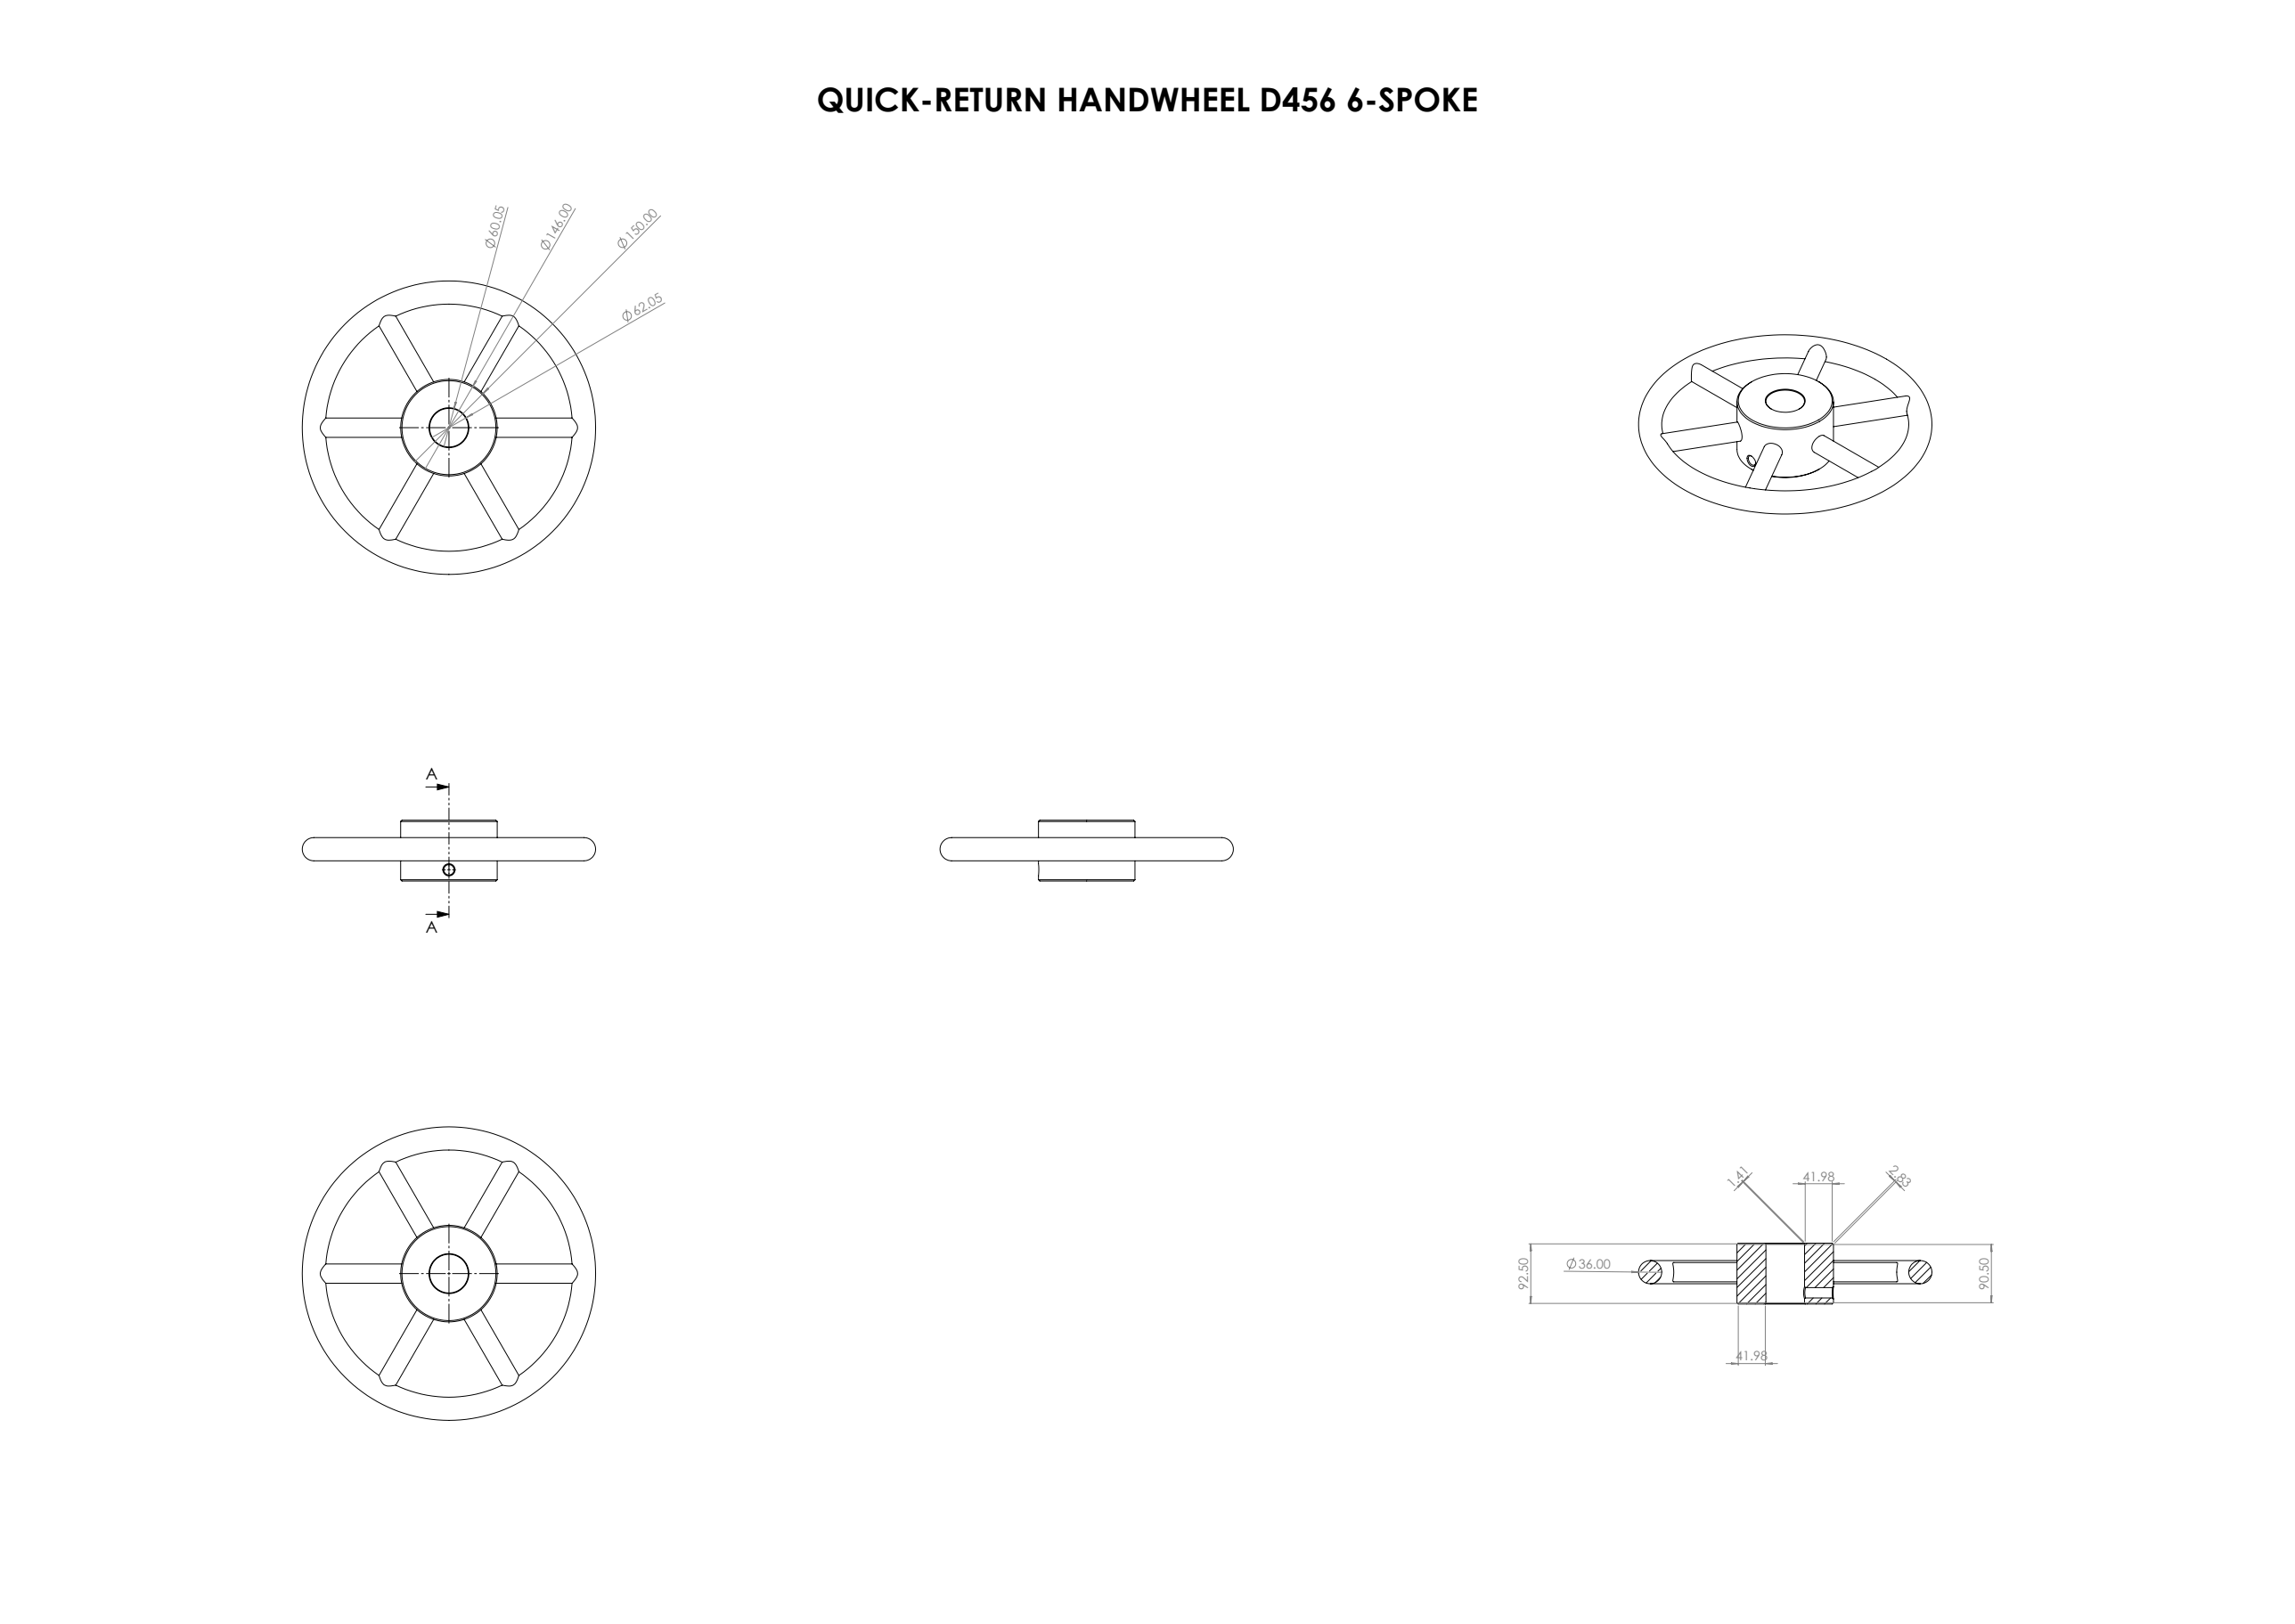
ISO-10303-21;
HEADER;
/* Generated by software containing ST-Developer
 * from STEP Tools, Inc. (www.steptools.com) 
 */

FILE_DESCRIPTION(
/* description */ (''),
/* implementation_level */ '2;1');

FILE_NAME(
/* name */ '07_Quick-Return_Handwheel_D456_6-Spoke.step',
/* time_stamp */ '2026-10-19T23:58:09-07:00',
/* author */ (''),
/* organization */ (''),
/* preprocessor_version */ 'ST-DEVELOPER v20.2',
/* originating_system */ 'Autodesk Translation Framework v15.15.0.0',
/* authorisation */ '');

FILE_SCHEMA (('AP203_CONFIGURATION_CONTROLLED_3D_DESIGN_OF_MECHANICAL_PARTS_AND_ASSEMBLIES_MIM_LF { 1 0 10303 203 3 1 4 }',
'AUTOMOTIVE_DESIGN { 1 0 10303 214 3 1 1 }','INTEGRATED_CNC_SCHEMA','MODEL_BASED_INTEGRATED_MANUFACTURING_SCHEMA',
'PROCESS_PLANNING_SCHEMA','AP242_MANAGED_MODEL_BASED_3D_ENGINEERING_MIM_LF { 1 0 10303 442 3 1 4 }'));
ENDSEC;

DATA;
#10=MECHANICAL_DESIGN_GEOMETRIC_PRESENTATION_REPRESENTATION('',(#411),#70757);
#142=TOROIDAL_SURFACE('',#27407,21.,1.8);
#272=B_SPLINE_SURFACE_WITH_KNOTS('',3,3,((#44072,#44073,#44074,#44075,#44076,
#44077,#44078,#44079,#44080,#44081,#44082,#44083,#44084,#44085,#44086,#44087,
#44088,#44089,#44090,#44091,#44092,#44093,#44094,#44095,#44096,#44097,#44098,
#44099,#44100,#44101,#44102,#44103,#44104,#44105,#44106,#44107,#44108,#44109,
#44110,#44111,#44112,#44113,#44114,#44115,#44116,#44117,#44118,#44119,#44120,
#44121,#44122,#44123,#44124,#44125,#44126,#44127,#44128,#44129,#44130,#44131,
#44132,#44133,#44134,#44135,#44136),(#44137,#44138,#44139,#44140,#44141,
#44142,#44143,#44144,#44145,#44146,#44147,#44148,#44149,#44150,#44151,#44152,
#44153,#44154,#44155,#44156,#44157,#44158,#44159,#44160,#44161,#44162,#44163,
#44164,#44165,#44166,#44167,#44168,#44169,#44170,#44171,#44172,#44173,#44174,
#44175,#44176,#44177,#44178,#44179,#44180,#44181,#44182,#44183,#44184,#44185,
#44186,#44187,#44188,#44189,#44190,#44191,#44192,#44193,#44194,#44195,#44196,
#44197,#44198,#44199,#44200,#44201),(#44202,#44203,#44204,#44205,#44206,
#44207,#44208,#44209,#44210,#44211,#44212,#44213,#44214,#44215,#44216,#44217,
#44218,#44219,#44220,#44221,#44222,#44223,#44224,#44225,#44226,#44227,#44228,
#44229,#44230,#44231,#44232,#44233,#44234,#44235,#44236,#44237,#44238,#44239,
#44240,#44241,#44242,#44243,#44244,#44245,#44246,#44247,#44248,#44249,#44250,
#44251,#44252,#44253,#44254,#44255,#44256,#44257,#44258,#44259,#44260,#44261,
#44262,#44263,#44264,#44265,#44266),(#44267,#44268,#44269,#44270,#44271,
#44272,#44273,#44274,#44275,#44276,#44277,#44278,#44279,#44280,#44281,#44282,
#44283,#44284,#44285,#44286,#44287,#44288,#44289,#44290,#44291,#44292,#44293,
#44294,#44295,#44296,#44297,#44298,#44299,#44300,#44301,#44302,#44303,#44304,
#44305,#44306,#44307,#44308,#44309,#44310,#44311,#44312,#44313,#44314,#44315,
#44316,#44317,#44318,#44319,#44320,#44321,#44322,#44323,#44324,#44325,#44326,
#44327,#44328,#44329,#44330,#44331)),.UNSPECIFIED.,.F.,.T.,.F.,(4,4),(4,
1,1,1,1,1,1,1,1,1,1,1,1,1,1,1,1,1,1,1,1,1,1,1,1,1,1,1,1,1,1,1,1,1,1,1,1,
1,1,1,1,1,1,1,1,1,1,1,1,1,1,1,1,1,1,1,1,1,1,1,1,1,4),(0.,1.),(0.,0.346838652723539,
0.433548315904424,0.455225731699645,0.476903147494867,0.498580563290088,
0.520257979085309,0.693677305447079,0.7153547212423,0.737032137037521,0.780386968627963,
0.823741800218406,0.867096631808848,0.953806294989733,0.997161126580175,
1.04051595817062,1.38735461089416,1.39096751352669,1.39458041615923,1.4018062214243,
1.41625783195445,1.42348363721953,1.4307094424846,1.44516105301475,1.50296749513534,
1.56077393725593,1.61858037937652,1.7341932636177,1.79199970573829,1.84980614785888,
2.08103191634124,2.13883835846183,2.19664480058242,2.25445124270301,2.31225768482359,
2.54348345330595,2.65909633754713,2.77470922178831,2.94812854815008,3.12154787451185,
3.20825753769274,3.29496720087362,3.38167686405451,3.42503169564495,3.43587040354256,
3.44670911144017,3.45754781933778,3.46838652723539,3.64180585359716,3.81522517995893,
3.85858001154937,3.90193484313982,3.9886445063207,4.07535416950159,4.11870900109203,
4.16206383268247,4.33548315904424,4.34632186694185,4.35716057483946,4.37883799063468,
4.42219282222513,4.50890248540601,4.85574113812955),.UNSPECIFIED.);
#273=B_SPLINE_SURFACE_WITH_KNOTS('',3,3,((#44815,#44816,#44817,#44818,#44819,
#44820,#44821,#44822,#44823,#44824,#44825,#44826,#44827,#44828,#44829,#44830,
#44831,#44832,#44833,#44834,#44835,#44836,#44837),(#44838,#44839,#44840,
#44841,#44842,#44843,#44844,#44845,#44846,#44847,#44848,#44849,#44850,#44851,
#44852,#44853,#44854,#44855,#44856,#44857,#44858,#44859,#44860),(#44861,
#44862,#44863,#44864,#44865,#44866,#44867,#44868,#44869,#44870,#44871,#44872,
#44873,#44874,#44875,#44876,#44877,#44878,#44879,#44880,#44881,#44882,#44883),
(#44884,#44885,#44886,#44887,#44888,#44889,#44890,#44891,#44892,#44893,
#44894,#44895,#44896,#44897,#44898,#44899,#44900,#44901,#44902,#44903,#44904,
#44905,#44906)),.UNSPECIFIED.,.F.,.T.,.F.,(4,4),(4,1,1,1,1,2,2,1,1,1,1,
1,2,1,1,1,1,4),(0.,1.),(1.16422336569995,1.62550842979414,2.08679349388834,
2.31743602593544,2.54807855798254,3.00936362207673,3.08125863299769,3.36971080227501,
3.65816297155233,3.73027601387166,3.802389056191,3.94661514082966,4.23506731010698,
4.71432612693143,5.19358494375588,5.67284376058034,5.91247316899256,6.15210257740479),
 .UNSPECIFIED.);
#381=SHAPE_REPRESENTATION_RELATIONSHIP('SRR','None',#70822,#396);
#396=ADVANCED_BREP_SHAPE_REPRESENTATION('',(#471),#70746);
#411=STYLED_ITEM('',(#71033),#471);
#471=MANIFOLD_SOLID_BREP('Handwheel',#26876);
#597=CYLINDRICAL_SURFACE('',#27400,0.805);
#598=CYLINDRICAL_SURFACE('',#27401,7.5);
#599=CYLINDRICAL_SURFACE('',#27404,3.0025);
#600=CYLINDRICAL_SURFACE('',#27416,1.49999999999999);
#601=CYLINDRICAL_SURFACE('',#27417,1.5);
#602=CYLINDRICAL_SURFACE('',#27418,1.5);
#603=CYLINDRICAL_SURFACE('',#27419,1.5);
#604=CYLINDRICAL_SURFACE('',#27420,1.5);
#605=CYLINDRICAL_SURFACE('',#27421,1.5);
#852=FACE_BOUND('',#4302,.T.);
#853=FACE_BOUND('',#4303,.T.);
#854=FACE_BOUND('',#4304,.T.);
#855=FACE_BOUND('',#4305,.T.);
#856=FACE_BOUND('',#4306,.T.);
#857=FACE_BOUND('',#4307,.T.);
#858=FACE_BOUND('',#4310,.T.);
#859=FACE_BOUND('',#4320,.T.);
#860=FACE_BOUND('',#4324,.T.);
#1102=B_SPLINE_CURVE_WITH_KNOTS('',3,(#44335,#44336,#44337,#44338,#44339,
#44340,#44341,#44342,#44343,#44344,#44345,#44346,#44347,#44348,#44349,#44350,
#44351,#44352,#44353,#44354,#44355,#44356,#44357,#44358,#44359,#44360,#44361,
#44362,#44363,#44364,#44365,#44366,#44367,#44368,#44369,#44370,#44371,#44372,
#44373,#44374,#44375,#44376,#44377,#44378,#44379,#44380,#44381,#44382,#44383,
#44384,#44385,#44386,#44387,#44388,#44389,#44390,#44391,#44392,#44393,#44394,
#44395,#44396,#44397,#44398,#44399),.UNSPECIFIED.,.T.,.F.,(4,1,1,1,1,1,
1,1,1,1,1,1,1,1,1,1,1,1,1,1,1,1,1,1,1,1,1,1,1,1,1,1,1,1,1,1,1,1,1,1,1,1,
1,1,1,1,1,1,1,1,1,1,1,1,1,1,1,1,1,1,1,1,4),(0.,0.346838652723539,0.433548315904424,
0.455225731699645,0.476903147494867,0.498580563290088,0.520257979085309,
0.693677305447079,0.7153547212423,0.737032137037521,0.780386968627963,0.823741800218406,
0.867096631808848,0.953806294989733,0.997161126580175,1.04051595817062,
1.38735461089416,1.39096751352669,1.39458041615923,1.4018062214243,1.41625783195445,
1.42348363721953,1.4307094424846,1.44516105301475,1.50296749513534,1.56077393725593,
1.61858037937652,1.7341932636177,1.79199970573829,1.84980614785888,2.08103191634124,
2.13883835846183,2.19664480058242,2.25445124270301,2.31225768482359,2.54348345330595,
2.65909633754713,2.77470922178831,2.94812854815008,3.12154787451185,3.20825753769274,
3.29496720087362,3.38167686405451,3.42503169564495,3.43587040354256,3.44670911144017,
3.45754781933778,3.46838652723539,3.64180585359716,3.81522517995893,3.85858001154937,
3.90193484313982,3.9886445063207,4.07535416950159,4.11870900109203,4.16206383268247,
4.33548315904424,4.34632186694185,4.35716057483946,4.37883799063468,4.42219282222513,
4.50890248540601,4.85574113812955),.UNSPECIFIED.);
#1103=B_SPLINE_CURVE_WITH_KNOTS('',3,(#44400,#44401,#44402,#44403,#44404,
#44405,#44406,#44407,#44408,#44409,#44410,#44411,#44412,#44413,#44414,#44415,
#44416,#44417,#44418,#44419,#44420,#44421,#44422,#44423,#44424,#44425,#44426,
#44427,#44428,#44429,#44430,#44431,#44432,#44433,#44434,#44435,#44436,#44437,
#44438,#44439,#44440,#44441,#44442,#44443,#44444,#44445,#44446,#44447,#44448,
#44449,#44450,#44451,#44452,#44453,#44454,#44455,#44456,#44457,#44458,#44459,
#44460,#44461,#44462,#44463,#44464),.UNSPECIFIED.,.T.,.F.,(4,1,1,1,1,1,
1,1,1,1,1,1,1,1,1,1,1,1,1,1,1,1,1,1,1,1,1,1,1,1,1,1,1,1,1,1,1,1,1,1,1,1,
1,1,1,1,1,1,1,1,1,1,1,1,1,1,1,1,1,1,1,1,4),(-4.85574113812955,-4.50890248540601,
-4.42219282222513,-4.37883799063468,-4.35716057483946,-4.34632186694185,
-4.33548315904424,-4.16206383268247,-4.11870900109203,-4.07535416950159,
-3.9886445063207,-3.90193484313982,-3.85858001154937,-3.81522517995893,
-3.64180585359716,-3.46838652723539,-3.45754781933778,-3.44670911144017,
-3.43587040354256,-3.42503169564495,-3.38167686405451,-3.29496720087362,
-3.20825753769274,-3.12154787451185,-2.94812854815008,-2.77470922178831,
-2.65909633754713,-2.54348345330595,-2.31225768482359,-2.25445124270301,
-2.19664480058242,-2.13883835846183,-2.08103191634124,-1.84980614785888,
-1.79199970573829,-1.7341932636177,-1.61858037937652,-1.56077393725593,
-1.50296749513534,-1.44516105301475,-1.4307094424846,-1.42348363721953,
-1.41625783195445,-1.4018062214243,-1.39458041615923,-1.39096751352669,
-1.38735461089416,-1.04051595817062,-0.997161126580175,-0.953806294989733,
-0.867096631808848,-0.823741800218406,-0.780386968627963,-0.737032137037521,
-0.7153547212423,-0.693677305447079,-0.520257979085309,-0.498580563290088,
-0.476903147494867,-0.455225731699645,-0.433548315904424,-0.346838652723539,
0.),.UNSPECIFIED.);
#1104=B_SPLINE_CURVE_WITH_KNOTS('',3,(#44468,#44469,#44470,#44471,#44472,
#44473,#44474,#44475,#44476,#44477,#44478,#44479,#44480,#44481,#44482,#44483,
#44484,#44485,#44486,#44487),.UNSPECIFIED.,.F.,.F.,(4,1,1,1,1,2,2,1,1,1,
1,1,2,1,4),(1.16422336569995,1.62550842979414,2.08679349388834,2.31743602593544,
2.54807855798254,3.00936362207673,3.08125863299769,3.36971080227501,3.65816297155233,
3.73027601387166,3.802389056191,3.94661514082966,4.23506731010698,4.71432612693143,
4.89579080658336),.UNSPECIFIED.);
#1105=B_SPLINE_CURVE_WITH_KNOTS('',3,(#44488,#44489,#44490,#44491,#44492,
#44493,#44494),.UNSPECIFIED.,.F.,.F.,(4,1,1,1,4),(4.89579080658336,5.19358494375588,
5.67284376058034,5.91247316899256,6.15210257740479),.UNSPECIFIED.);
#1106=B_SPLINE_CURVE_WITH_KNOTS('',3,(#44502,#44503,#44504,#44505,#44506,
#44507,#44508,#44509,#44510,#44511,#44512,#44513,#44514,#44515,#44516,#44517,
#44518,#44519,#44520,#44521,#44522,#44523,#44524,#44525,#44526,#44527),
 .UNSPECIFIED.,.F.,.F.,(4,2,2,2,2,2,2,2,2,2,2,2,4),(2.26670802646318,2.55003859116132,
2.83336915585947,3.40003028525577,3.96672316909106,4.25006961100871,4.53341605292635,
4.816762494844,5.10010893676165,5.66680182059694,6.23346294999324,6.51679351469138,
6.80012407938953),.UNSPECIFIED.);
#1107=B_SPLINE_CURVE_WITH_KNOTS('',3,(#44532,#44533,#44534,#44535,#44536,
#44537,#44538,#44539,#44540,#44541,#44542,#44543,#44544,#44545),
 .UNSPECIFIED.,.F.,.F.,(4,2,2,2,2,2,4),(6.80012407938953,7.08345464408768,
7.36678520878583,7.93344633818212,8.50013922201742,8.78348566393506,9.06683210585271),
 .UNSPECIFIED.);
#1108=B_SPLINE_CURVE_WITH_KNOTS('',3,(#44546,#44547,#44548,#44549,#44550,
#44551,#44552,#44553,#44554,#44555,#44556,#44557,#44558,#44559),
 .UNSPECIFIED.,.F.,.F.,(4,2,2,2,2,2,4),(0.,0.283346441917647,0.566692883835293,
1.13338576767059,1.70004689706688,1.98337746176503,2.26670802646318),
 .UNSPECIFIED.);
#1109=B_SPLINE_CURVE_WITH_KNOTS('',3,(#44561,#44562,#44563,#44564,#44565,
#44566,#44567,#44568,#44569,#44570,#44571,#44572,#44573,#44574,#44575,#44576,
#44577,#44578,#44579,#44580,#44581,#44582,#44583,#44584,#44585,#44586,#44587,
#44588,#44589,#44590,#44591,#44592,#44593,#44594,#44595,#44596,#44597,#44598,
#44599,#44600,#44601,#44602,#44603,#44604,#44605,#44606,#44607,#44608,#44609,
#44610),.UNSPECIFIED.,.T.,.F.,(4,2,2,2,2,2,2,2,2,2,2,2,2,2,2,2,2,2,2,2,
2,2,2,2,4),(0.,0.283346441917647,0.566692883835293,1.13338576767059,1.70004689706688,
1.98337746176503,2.26670802646318,2.55003859116132,2.83336915585947,3.40003028525577,
3.96672316909106,4.25006961100871,4.53341605292635,4.816762494844,5.10010893676165,
5.66680182059694,6.23346294999323,6.51679351469138,6.80012407938953,7.08345464408768,
7.36678520878582,7.93344633818212,8.50013922201741,8.78348566393506,9.06683210585271),
 .UNSPECIFIED.);
#1110=B_SPLINE_CURVE_WITH_KNOTS('',3,(#44612,#44613,#44614,#44615,#44616,
#44617,#44618,#44619,#44620,#44621,#44622,#44623,#44624,#44625,#44626,#44627,
#44628,#44629,#44630,#44631,#44632,#44633,#44634,#44635,#44636,#44637,#44638,
#44639,#44640,#44641,#44642,#44643,#44644,#44645,#44646,#44647,#44648,#44649,
#44650,#44651,#44652,#44653,#44654,#44655,#44656,#44657,#44658,#44659,#44660,
#44661),.UNSPECIFIED.,.T.,.F.,(4,2,2,2,2,2,2,2,2,2,2,2,2,2,2,2,2,2,2,2,
2,2,2,2,4),(0.,0.283346441917646,0.566692883835292,1.13338576767058,1.70004689706688,
1.98337746176503,2.26670802646318,2.55003859116133,2.83336915585948,3.40003028525578,
3.96672316909107,4.25006961100872,4.53341605292636,4.81676249484401,5.10010893676166,
5.66680182059695,6.23346294999325,6.5167935146914,6.80012407938955,7.0834546440877,
7.36678520878585,7.93344633818214,8.50013922201744,8.78348566393508,9.06683210585273),
 .UNSPECIFIED.);
#1111=B_SPLINE_CURVE_WITH_KNOTS('',3,(#44663,#44664,#44665,#44666,#44667,
#44668,#44669,#44670,#44671,#44672,#44673,#44674,#44675,#44676,#44677,#44678,
#44679,#44680,#44681,#44682,#44683,#44684,#44685,#44686,#44687,#44688,#44689,
#44690,#44691,#44692,#44693,#44694,#44695,#44696,#44697,#44698,#44699,#44700,
#44701,#44702,#44703,#44704,#44705,#44706,#44707,#44708,#44709,#44710,#44711,
#44712),.UNSPECIFIED.,.T.,.F.,(4,2,2,2,2,2,2,2,2,2,2,2,2,2,2,2,2,2,2,2,
2,2,2,2,4),(0.,0.283346441917645,0.566692883835289,1.13338576767058,1.70004689706688,
1.98337746176503,2.26670802646318,2.55003859116133,2.83336915585948,3.40003028525578,
3.96672316909107,4.25006961100871,4.53341605292636,4.816762494844,5.10010893676165,
5.66680182059694,6.23346294999324,6.51679351469139,6.80012407938954,7.08345464408769,
7.36678520878584,7.93344633818214,8.50013922201743,8.78348566393507,9.06683210585271),
 .UNSPECIFIED.);
#1112=B_SPLINE_CURVE_WITH_KNOTS('',3,(#44714,#44715,#44716,#44717,#44718,
#44719,#44720,#44721,#44722,#44723,#44724,#44725,#44726,#44727,#44728,#44729,
#44730,#44731,#44732,#44733,#44734,#44735,#44736,#44737,#44738,#44739,#44740,
#44741,#44742,#44743,#44744,#44745,#44746,#44747,#44748,#44749,#44750,#44751,
#44752,#44753,#44754,#44755,#44756,#44757,#44758,#44759,#44760,#44761,#44762,
#44763),.UNSPECIFIED.,.T.,.F.,(4,2,2,2,2,2,2,2,2,2,2,2,2,2,2,2,2,2,2,2,
2,2,2,2,4),(0.,0.283346441917645,0.566692883835291,1.13338576767058,1.70004689706688,
1.98337746176503,2.26670802646318,2.55003859116133,2.83336915585948,3.40003028525578,
3.96672316909107,4.25006961100872,4.53341605292636,4.81676249484401,5.10010893676165,
5.66680182059694,6.23346294999324,6.51679351469139,6.80012407938954,7.08345464408769,
7.36678520878584,7.93344633818214,8.50013922201743,8.78348566393508,9.06683210585273),
 .UNSPECIFIED.);
#1113=B_SPLINE_CURVE_WITH_KNOTS('',3,(#44765,#44766,#44767,#44768,#44769,
#44770,#44771,#44772,#44773,#44774,#44775,#44776,#44777,#44778,#44779,#44780,
#44781,#44782,#44783,#44784,#44785,#44786,#44787,#44788,#44789,#44790,#44791,
#44792,#44793,#44794,#44795,#44796,#44797,#44798,#44799,#44800,#44801,#44802,
#44803,#44804,#44805,#44806,#44807,#44808,#44809,#44810,#44811,#44812,#44813,
#44814),.UNSPECIFIED.,.T.,.F.,(4,2,2,2,2,2,2,2,2,2,2,2,2,2,2,2,2,2,2,2,
2,2,2,2,4),(0.,0.283346441917644,0.566692883835287,1.13338576767057,1.70004689706687,
1.98337746176502,2.26670802646317,2.55003859116132,2.83336915585947,3.40003028525577,
3.96672316909106,4.2500696110087,4.53341605292635,4.81676249484399,5.10010893676164,
5.66680182059692,6.23346294999322,6.51679351469137,6.80012407938952,7.08345464408767,
7.36678520878582,7.93344633818212,8.50013922201741,8.78348566393505,9.0668321058527),
 .UNSPECIFIED.);
#1114=B_SPLINE_CURVE_WITH_KNOTS('',3,(#44910,#44911,#44912,#44913,#44914,
#44915,#44916,#44917,#44918,#44919),.UNSPECIFIED.,.F.,.F.,(4,1,1,1,1,2,
4),(-6.15210257740479,-5.91247316899256,-5.67284376058034,-5.19358494375588,
-4.71432612693143,-4.23506731010698,-4.12936945995859),.UNSPECIFIED.);
#1115=B_SPLINE_CURVE_WITH_KNOTS('',3,(#44921,#44922,#44923,#44924,#44925,
#44926,#44927,#44928,#44929),.UNSPECIFIED.,.F.,.F.,(4,1,1,1,1,1,4),(-4.12936945995859,
-3.94661514082966,-3.802389056191,-3.73027601387166,-3.65816297155233,-3.36971080227501,
-3.18695648314609),.UNSPECIFIED.);
#1116=B_SPLINE_CURVE_WITH_KNOTS('',3,(#44930,#44931,#44932,#44933,#44934,
#44935,#44936,#44937,#44938,#44939,#44940,#44941),.UNSPECIFIED.,.F.,.F.,
(4,2,2,1,1,1,1,4),(-3.18695648314609,-3.08125863299769,-3.00936362207673,
-2.54807855798254,-2.31743602593544,-2.08679349388834,-1.62550842979414,
-1.16422336569995),.UNSPECIFIED.);
#1117=B_SPLINE_CURVE_WITH_KNOTS('',3,(#44954,#44955,#44956,#44957,#44958,
#44959,#44960,#44961,#44962,#44963,#44964,#44965,#44966,#44967,#44968,#44969,
#44970,#44971,#44972,#44973,#44974,#44975,#44976,#44977,#44978,#44979),
 .UNSPECIFIED.,.F.,.F.,(4,2,2,2,2,2,2,2,2,2,2,2,4),(2.38843711110425,2.73991717768157,
3.18290676087182,3.79372965899082,4.41467175444456,4.65907472712817,4.82558871054652,
5.00595266090074,5.33402028952842,5.78028507040623,6.42716241421292,6.9078895490275,
7.2160083509484),.UNSPECIFIED.);
#1118=B_SPLINE_CURVE_WITH_KNOTS('',3,(#44983,#44984,#44985,#44986,#44987,
#44988,#44989,#44990,#44991,#44992,#44993,#44994,#44995,#44996,#44997,#44998,
#44999,#45000,#45001,#45002,#45003,#45004,#45005,#45006),.UNSPECIFIED.,
 .F.,.F.,(4,2,2,2,2,2,2,2,2,2,2,4),(2.22240766759392,2.51631391142046,2.86860433098781,
3.30769808976926,3.80274376109231,4.15490018438336,4.49463257862064,4.88220060274562,
5.47385284067091,6.01546654165425,6.42750720918413,6.5614735041056),
 .UNSPECIFIED.);
#1119=B_SPLINE_CURVE_WITH_KNOTS('',3,(#45010,#45011,#45012,#45013,#45014,
#45015,#45016,#45017,#45018,#45019,#45020,#45021,#45022,#45023,#45024,#45025,
#45026,#45027,#45028,#45029,#45030,#45031,#45032,#45033,#45034,#45035),
 .UNSPECIFIED.,.F.,.F.,(4,2,2,2,2,2,2,2,2,2,2,2,4),(2.38843711109743,2.73991717767369,
3.18290676086253,3.79372965898107,4.41467175443591,4.65907472712015,4.82558871053879,
5.00595266089327,5.33402028952175,5.78028507040088,6.42716241420991,6.90788954902662,
7.216008350949),.UNSPECIFIED.);
#1120=B_SPLINE_CURVE_WITH_KNOTS('',3,(#45039,#45040,#45041,#45042,#45043,
#45044,#45045,#45046,#45047,#45048,#45049,#45050,#45051,#45052,#45053,#45054,
#45055,#45056,#45057,#45058,#45059,#45060,#45061,#45062,#45063,#45064),
 .UNSPECIFIED.,.F.,.F.,(4,2,2,2,2,2,2,2,2,2,2,2,4),(2.3884371111015,2.73991717767853,
3.18290676086844,3.79372965898921,4.41467175444667,4.65907472713178,4.82558871055129,
5.00595266090689,5.33402028953752,5.7802850704188,6.4271624142303,6.90788954904922,
7.21600835097295),.UNSPECIFIED.);
#1121=B_SPLINE_CURVE_WITH_KNOTS('',3,(#45068,#45069,#45070,#45071,#45072,
#45073,#45074,#45075,#45076,#45077,#45078,#45079,#45080,#45081,#45082,#45083,
#45084,#45085,#45086,#45087,#45088,#45089,#45090,#45091),.UNSPECIFIED.,
 .F.,.F.,(4,2,2,2,2,2,2,2,2,2,2,4),(2.2224076675936,2.51631391142003,2.8686043309871,
3.30769808976771,3.80274376108999,4.15490018438039,4.49463257861656,4.88220060273995,
5.47385284066319,6.01546654164533,6.42750720917386,6.56147350409479),
 .UNSPECIFIED.);
#1122=B_SPLINE_CURVE_WITH_KNOTS('',3,(#45095,#45096,#45097,#45098,#45099,
#45100,#45101,#45102,#45103,#45104,#45105,#45106,#45107,#45108,#45109,#45110,
#45111,#45112,#45113,#45114,#45115,#45116,#45117,#45118,#45119,#45120),
 .UNSPECIFIED.,.F.,.F.,(4,2,2,2,2,2,2,2,2,2,2,2,4),(2.38843711111166,2.73991717769056,
3.18290676088307,3.79372965900683,4.4146717544666,4.65907472715359,4.82558871057392,
5.00595266093029,5.33402028956311,5.78028507044741,6.42716241426385,6.90788954908701,
7.21600835101346),.UNSPECIFIED.);
#1123=B_SPLINE_CURVE_WITH_KNOTS('',3,(#45123,#45124,#45125,#45126,#45127,
#45128,#45129,#45130,#45131,#45132,#45133,#45134,#45135,#45136,#45137,#45138),
 .UNSPECIFIED.,.F.,.F.,(4,2,2,2,2,2,2,4),(0.,0.163315076677852,0.428209466619433,
0.780925001042535,1.38907330894996,1.92592908231006,2.3460116526462,2.38843711111166),
 .UNSPECIFIED.);
#1124=B_SPLINE_CURVE_WITH_KNOTS('',3,(#45139,#45140,#45141,#45142,#45143,
#45144,#45145,#45146,#45147,#45148,#45149,#45150,#45151,#45152,#45153,#45154),
 .UNSPECIFIED.,.F.,.F.,(4,2,2,2,2,2,2,4),(7.21600835101346,7.31138807064545,
7.71016155437429,8.19219414711906,8.90541863857944,9.32049440063031,9.51422700130749,
9.59086664090117),.UNSPECIFIED.);
#1125=B_SPLINE_CURVE_WITH_KNOTS('',3,(#45156,#45157,#45158,#45159,#45160,
#45161,#45162,#45163,#45164,#45165,#45166,#45167,#45168,#45169),
 .UNSPECIFIED.,.F.,.F.,(4,2,2,2,2,2,4),(0.,0.314217231275812,0.709389217563233,
1.32114854838333,1.80769659482899,2.17854969785705,2.2224076675936),
 .UNSPECIFIED.);
#1126=B_SPLINE_CURVE_WITH_KNOTS('',3,(#45170,#45171,#45172,#45173,#45174,
#45175,#45176,#45177,#45178,#45179,#45180,#45181,#45182,#45183),
 .UNSPECIFIED.,.F.,.F.,(4,2,2,2,2,2,4),(6.56147350409479,6.79183498105132,
7.15166374851714,7.58660248971605,8.17287181265779,8.55036069386147,8.66642098576321),
 .UNSPECIFIED.);
#1127=B_SPLINE_CURVE_WITH_KNOTS('',3,(#45185,#45186,#45187,#45188,#45189,
#45190,#45191,#45192,#45193,#45194,#45195,#45196,#45197,#45198,#45199,#45200),
 .UNSPECIFIED.,.F.,.F.,(4,2,2,2,2,2,2,4),(0.,0.163315076677636,0.428209466618054,
0.780925001039408,1.38907330894433,1.92592908230217,2.34601165263628,2.3884371111015),
 .UNSPECIFIED.);
#1128=B_SPLINE_CURVE_WITH_KNOTS('',3,(#45201,#45202,#45203,#45204,#45205,
#45206,#45207,#45208,#45209,#45210,#45211,#45212,#45213,#45214,#45215,#45216),
 .UNSPECIFIED.,.F.,.F.,(4,2,2,2,2,2,2,4),(7.21600835097295,7.311388070604,
7.71016155432903,8.19219414706878,8.90541863852133,9.32049440056781,9.51422700124278,
9.59086664083621),.UNSPECIFIED.);
#1129=B_SPLINE_CURVE_WITH_KNOTS('',3,(#45218,#45219,#45220,#45221,#45222,
#45223,#45224,#45225,#45226,#45227,#45228,#45229,#45230,#45231,#45232,#45233),
 .UNSPECIFIED.,.F.,.F.,(4,2,2,2,2,2,2,4),(0.,0.163315076677541,0.428209466617523,
0.780925001038301,1.38907330894207,1.92592908229898,2.34601165263229,2.38843711109743),
 .UNSPECIFIED.);
#1130=B_SPLINE_CURVE_WITH_KNOTS('',3,(#45234,#45235,#45236,#45237,#45238,
#45239,#45240,#45241,#45242,#45243,#45244,#45245,#45246,#45247,#45248,#45249),
 .UNSPECIFIED.,.F.,.F.,(4,2,2,2,2,2,2,4),(7.216008350949,7.31138807057958,
7.71016155430275,8.19219414704005,8.90541863848882,9.32049440053308,9.51422700120671,
9.59086664079997),.UNSPECIFIED.);
#1131=B_SPLINE_CURVE_WITH_KNOTS('',3,(#45251,#45252,#45253,#45254,#45255,
#45256,#45257,#45258,#45259,#45260,#45261,#45262,#45263,#45264),
 .UNSPECIFIED.,.F.,.F.,(4,2,2,2,2,2,4),(0.,0.314217231275878,0.709389217563644,
1.3211485483838,1.80769659482918,2.1785496978573,2.22240766759392),
 .UNSPECIFIED.);
#1132=B_SPLINE_CURVE_WITH_KNOTS('',3,(#45265,#45266,#45267,#45268,#45269,
#45270,#45271,#45272,#45273,#45274,#45275,#45276,#45277,#45278),
 .UNSPECIFIED.,.F.,.F.,(4,2,2,2,2,2,4),(6.5614735041056,6.79183498106296,
7.15166374853013,7.58660248973094,8.17287181267555,8.5503606938791,8.66642098578064),
 .UNSPECIFIED.);
#1133=B_SPLINE_CURVE_WITH_KNOTS('',3,(#45280,#45281,#45282,#45283,#45284,
#45285,#45286,#45287,#45288,#45289,#45290,#45291,#45292,#45293,#45294,#45295),
 .UNSPECIFIED.,.F.,.F.,(4,2,2,2,2,2,2,4),(0.,0.163315076677694,0.428209466618468,
0.780925001040192,1.38907330894576,1.92592908230429,2.34601165263891,2.38843711110425),
 .UNSPECIFIED.);
#1134=B_SPLINE_CURVE_WITH_KNOTS('',3,(#45296,#45297,#45298,#45299,#45300,
#45301,#45302,#45303,#45304,#45305,#45306,#45307,#45308,#45309,#45310,#45311),
 .UNSPECIFIED.,.F.,.F.,(4,2,2,2,2,2,2,4),(7.2160083509484,7.31138807057855,
7.71016155429981,8.1921941470349,8.90541863848042,9.3204944005228,9.5142270011958,
9.59086664078899),.UNSPECIFIED.);
#1763=PLANE('',#27424);
#1764=PLANE('',#27429);
#2803=FACE_OUTER_BOUND('',#4299,.T.);
#2804=FACE_OUTER_BOUND('',#4300,.T.);
#2805=FACE_OUTER_BOUND('',#4301,.T.);
#2806=FACE_OUTER_BOUND('',#4308,.T.);
#2807=FACE_OUTER_BOUND('',#4309,.T.);
#2808=FACE_OUTER_BOUND('',#4311,.T.);
#2809=FACE_OUTER_BOUND('',#4312,.T.);
#2810=FACE_OUTER_BOUND('',#4313,.T.);
#2811=FACE_OUTER_BOUND('',#4314,.T.);
#2812=FACE_OUTER_BOUND('',#4315,.T.);
#2813=FACE_OUTER_BOUND('',#4316,.T.);
#2814=FACE_OUTER_BOUND('',#4317,.T.);
#2815=FACE_OUTER_BOUND('',#4318,.T.);
#2816=FACE_OUTER_BOUND('',#4319,.T.);
#2817=FACE_OUTER_BOUND('',#4321,.T.);
#2818=FACE_OUTER_BOUND('',#4322,.T.);
#2819=FACE_OUTER_BOUND('',#4323,.T.);
#2820=FACE_OUTER_BOUND('',#4325,.T.);
#4299=EDGE_LOOP('',(#18760,#18761,#18762,#18763));
#4300=EDGE_LOOP('',(#18764,#18765,#18766,#18767,#18768));
#4301=EDGE_LOOP('',(#18769,#18770,#18771,#18772,#18773,#18774,#18775,#18776,
#18777));
#4302=EDGE_LOOP('',(#18778));
#4303=EDGE_LOOP('',(#18779));
#4304=EDGE_LOOP('',(#18780));
#4305=EDGE_LOOP('',(#18781));
#4306=EDGE_LOOP('',(#18782));
#4307=EDGE_LOOP('',(#18783));
#4308=EDGE_LOOP('',(#18784,#18785,#18786,#18787,#18788,#18789,#18790));
#4309=EDGE_LOOP('',(#18791,#18792,#18793,#18794));
#4310=EDGE_LOOP('',(#18795,#18796,#18797));
#4311=EDGE_LOOP('',(#18798,#18799,#18800,#18801,#18802,#18803,#18804,#18805,
#18806,#18807,#18808,#18809,#18810,#18811,#18812,#18813,#18814,#18815,#18816,
#18817,#18818,#18819,#18820,#18821,#18822,#18823,#18824,#18825,#18826,#18827,
#18828,#18829,#18830,#18831));
#4312=EDGE_LOOP('',(#18832,#18833,#18834,#18835,#18836,#18837));
#4313=EDGE_LOOP('',(#18838,#18839,#18840,#18841,#18842,#18843));
#4314=EDGE_LOOP('',(#18844,#18845,#18846,#18847,#18848,#18849,#18850,#18851));
#4315=EDGE_LOOP('',(#18852,#18853,#18854,#18855,#18856,#18857));
#4316=EDGE_LOOP('',(#18858,#18859,#18860,#18861,#18862,#18863));
#4317=EDGE_LOOP('',(#18864,#18865,#18866,#18867,#18868,#18869));
#4318=EDGE_LOOP('',(#18870,#18871,#18872,#18873));
#4319=EDGE_LOOP('',(#18874));
#4320=EDGE_LOOP('',(#18875));
#4321=EDGE_LOOP('',(#18876,#18877,#18878,#18879));
#4322=EDGE_LOOP('',(#18880,#18881,#18882,#18883));
#4323=EDGE_LOOP('',(#18884));
#4324=EDGE_LOOP('',(#18885));
#4325=EDGE_LOOP('',(#18886,#18887,#18888,#18889));
#5908=LINE('',#44334,#8405);
#5909=LINE('',#44495,#8406);
#5910=LINE('',#44500,#8407);
#5911=LINE('',#44529,#8408);
#5912=LINE('',#44908,#8409);
#5913=LINE('',#44946,#8410);
#5914=LINE('',#45313,#8411);
#5915=LINE('',#45315,#8412);
#5916=LINE('',#45317,#8413);
#5917=LINE('',#45319,#8414);
#5918=LINE('',#45321,#8415);
#5919=LINE('',#45323,#8416);
#5920=LINE('',#45326,#8417);
#5921=LINE('',#45332,#8418);
#5922=LINE('',#45336,#8419);
#5923=LINE('',#45341,#8420);
#8405=VECTOR('',#29957,1.);
#8406=VECTOR('',#29960,0.805);
#8407=VECTOR('',#29965,7.5);
#8408=VECTOR('',#29966,7.5);
#8409=VECTOR('',#29969,1.);
#8410=VECTOR('',#29974,3.0025);
#8411=VECTOR('',#29997,1.49999999999999);
#8412=VECTOR('',#30000,1.5);
#8413=VECTOR('',#30003,1.5);
#8414=VECTOR('',#30006,1.5);
#8415=VECTOR('',#30009,1.5);
#8416=VECTOR('',#30012,1.5);
#8417=VECTOR('',#30015,3.0525);
#8418=VECTOR('',#30024,7.4);
#8419=VECTOR('',#30029,7.4);
#8420=VECTOR('',#30036,3.0525);
#10770=CIRCLE('',#27402,7.5);
#10771=CIRCLE('',#27403,7.5);
#10772=CIRCLE('',#27405,3.0025);
#10773=CIRCLE('',#27406,3.0025);
#10774=CIRCLE('',#27408,1.8);
#10775=CIRCLE('',#27409,19.2);
#10776=CIRCLE('',#27410,19.2);
#10777=CIRCLE('',#27411,19.2);
#10778=CIRCLE('',#27412,19.2);
#10779=CIRCLE('',#27413,19.2);
#10780=CIRCLE('',#27414,19.2);
#10781=CIRCLE('',#27415,19.2);
#10782=CIRCLE('',#27423,3.1025);
#10783=CIRCLE('',#27425,7.3);
#10784=CIRCLE('',#27428,7.3);
#10785=CIRCLE('',#27430,3.1025);
#11550=VERTEX_POINT('',#44332);
#11551=VERTEX_POINT('',#44333);
#11552=VERTEX_POINT('',#44466);
#11553=VERTEX_POINT('',#44467);
#11554=VERTEX_POINT('',#44497);
#11555=VERTEX_POINT('',#44499);
#11556=VERTEX_POINT('',#44501);
#11557=VERTEX_POINT('',#44528);
#11558=VERTEX_POINT('',#44531);
#11559=VERTEX_POINT('',#44560);
#11560=VERTEX_POINT('',#44611);
#11561=VERTEX_POINT('',#44662);
#11562=VERTEX_POINT('',#44713);
#11563=VERTEX_POINT('',#44764);
#11564=VERTEX_POINT('',#44907);
#11565=VERTEX_POINT('',#44909);
#11566=VERTEX_POINT('',#44920);
#11567=VERTEX_POINT('',#44943);
#11568=VERTEX_POINT('',#44945);
#11569=VERTEX_POINT('',#44949);
#11570=VERTEX_POINT('',#44951);
#11571=VERTEX_POINT('',#44953);
#11572=VERTEX_POINT('',#44980);
#11573=VERTEX_POINT('',#44982);
#11574=VERTEX_POINT('',#45007);
#11575=VERTEX_POINT('',#45009);
#11576=VERTEX_POINT('',#45036);
#11577=VERTEX_POINT('',#45038);
#11578=VERTEX_POINT('',#45065);
#11579=VERTEX_POINT('',#45067);
#11580=VERTEX_POINT('',#45092);
#11581=VERTEX_POINT('',#45094);
#11582=VERTEX_POINT('',#45122);
#11583=VERTEX_POINT('',#45155);
#11584=VERTEX_POINT('',#45184);
#11585=VERTEX_POINT('',#45217);
#11586=VERTEX_POINT('',#45250);
#11587=VERTEX_POINT('',#45279);
#11588=VERTEX_POINT('',#45325);
#11589=VERTEX_POINT('',#45329);
#11590=VERTEX_POINT('',#45334);
#11591=VERTEX_POINT('',#45338);
#14233=EDGE_CURVE('',#11550,#11551,#5908,.T.);
#14234=EDGE_CURVE('',#11551,#11551,#1102,.T.);
#14235=EDGE_CURVE('',#11550,#11550,#1103,.T.);
#14236=EDGE_CURVE('',#11552,#11553,#1104,.T.);
#14237=EDGE_CURVE('',#11553,#11552,#1105,.T.);
#14238=EDGE_CURVE('',#11553,#11551,#5909,.T.);
#14239=EDGE_CURVE('',#11554,#11554,#10770,.T.);
#14240=EDGE_CURVE('',#11554,#11555,#5910,.T.);
#14241=EDGE_CURVE('',#11555,#11556,#1106,.T.);
#14242=EDGE_CURVE('',#11556,#11557,#5911,.T.);
#14243=EDGE_CURVE('',#11557,#11557,#10771,.T.);
#14244=EDGE_CURVE('',#11556,#11558,#1107,.T.);
#14245=EDGE_CURVE('',#11558,#11555,#1108,.T.);
#14246=EDGE_CURVE('',#11559,#11559,#1109,.T.);
#14247=EDGE_CURVE('',#11560,#11560,#1110,.T.);
#14248=EDGE_CURVE('',#11561,#11561,#1111,.T.);
#14249=EDGE_CURVE('',#11562,#11562,#1112,.T.);
#14250=EDGE_CURVE('',#11563,#11563,#1113,.T.);
#14251=EDGE_CURVE('',#11564,#11552,#5912,.T.);
#14252=EDGE_CURVE('',#11564,#11565,#1114,.T.);
#14253=EDGE_CURVE('',#11565,#11566,#1115,.T.);
#14254=EDGE_CURVE('',#11566,#11564,#1116,.T.);
#14255=EDGE_CURVE('',#11567,#11567,#10772,.T.);
#14256=EDGE_CURVE('',#11567,#11568,#5913,.T.);
#14257=EDGE_CURVE('',#11568,#11568,#10773,.T.);
#14258=EDGE_CURVE('',#11569,#11569,#10774,.T.);
#14259=EDGE_CURVE('',#11570,#11569,#10775,.T.);
#14260=EDGE_CURVE('',#11571,#11570,#1117,.T.);
#14261=EDGE_CURVE('',#11572,#11571,#10776,.T.);
#14262=EDGE_CURVE('',#11573,#11572,#1118,.T.);
#14263=EDGE_CURVE('',#11574,#11573,#10777,.T.);
#14264=EDGE_CURVE('',#11575,#11574,#1119,.T.);
#14265=EDGE_CURVE('',#11576,#11575,#10778,.T.);
#14266=EDGE_CURVE('',#11577,#11576,#1120,.T.);
#14267=EDGE_CURVE('',#11578,#11577,#10779,.T.);
#14268=EDGE_CURVE('',#11579,#11578,#1121,.T.);
#14269=EDGE_CURVE('',#11580,#11579,#10780,.T.);
#14270=EDGE_CURVE('',#11581,#11580,#1122,.T.);
#14271=EDGE_CURVE('',#11569,#11581,#10781,.T.);
#14272=EDGE_CURVE('',#11582,#11581,#1123,.T.);
#14273=EDGE_CURVE('',#11580,#11582,#1124,.T.);
#14274=EDGE_CURVE('',#11583,#11579,#1125,.T.);
#14275=EDGE_CURVE('',#11578,#11583,#1126,.T.);
#14276=EDGE_CURVE('',#11584,#11577,#1127,.T.);
#14277=EDGE_CURVE('',#11576,#11584,#1128,.T.);
#14278=EDGE_CURVE('',#11585,#11575,#1129,.T.);
#14279=EDGE_CURVE('',#11574,#11585,#1130,.T.);
#14280=EDGE_CURVE('',#11586,#11573,#1131,.T.);
#14281=EDGE_CURVE('',#11572,#11586,#1132,.T.);
#14282=EDGE_CURVE('',#11587,#11571,#1133,.T.);
#14283=EDGE_CURVE('',#11570,#11587,#1134,.T.);
#14284=EDGE_CURVE('',#11563,#11576,#5914,.T.);
#14285=EDGE_CURVE('',#11562,#11574,#5915,.T.);
#14286=EDGE_CURVE('',#11558,#11572,#5916,.T.);
#14287=EDGE_CURVE('',#11561,#11570,#5917,.T.);
#14288=EDGE_CURVE('',#11560,#11580,#5918,.T.);
#14289=EDGE_CURVE('',#11559,#11578,#5919,.T.);
#14290=EDGE_CURVE('',#11568,#11588,#5920,.T.);
#14291=EDGE_CURVE('',#11588,#11588,#10782,.T.);
#14292=EDGE_CURVE('',#11589,#11589,#10783,.T.);
#14293=EDGE_CURVE('',#11557,#11589,#5921,.T.);
#14294=EDGE_CURVE('',#11590,#11590,#10784,.T.);
#14295=EDGE_CURVE('',#11590,#11554,#5922,.T.);
#14296=EDGE_CURVE('',#11591,#11591,#10785,.T.);
#14297=EDGE_CURVE('',#11591,#11567,#5923,.T.);
#18760=ORIENTED_EDGE('',*,*,#14233,.T.);
#18761=ORIENTED_EDGE('',*,*,#14234,.T.);
#18762=ORIENTED_EDGE('',*,*,#14233,.F.);
#18763=ORIENTED_EDGE('',*,*,#14235,.T.);
#18764=ORIENTED_EDGE('',*,*,#14236,.F.);
#18765=ORIENTED_EDGE('',*,*,#14237,.F.);
#18766=ORIENTED_EDGE('',*,*,#14238,.T.);
#18767=ORIENTED_EDGE('',*,*,#14234,.F.);
#18768=ORIENTED_EDGE('',*,*,#14238,.F.);
#18769=ORIENTED_EDGE('',*,*,#14239,.F.);
#18770=ORIENTED_EDGE('',*,*,#14240,.T.);
#18771=ORIENTED_EDGE('',*,*,#14241,.T.);
#18772=ORIENTED_EDGE('',*,*,#14242,.T.);
#18773=ORIENTED_EDGE('',*,*,#14243,.T.);
#18774=ORIENTED_EDGE('',*,*,#14242,.F.);
#18775=ORIENTED_EDGE('',*,*,#14244,.T.);
#18776=ORIENTED_EDGE('',*,*,#14245,.T.);
#18777=ORIENTED_EDGE('',*,*,#14240,.F.);
#18778=ORIENTED_EDGE('',*,*,#14246,.T.);
#18779=ORIENTED_EDGE('',*,*,#14247,.T.);
#18780=ORIENTED_EDGE('',*,*,#14248,.T.);
#18781=ORIENTED_EDGE('',*,*,#14249,.T.);
#18782=ORIENTED_EDGE('',*,*,#14250,.T.);
#18783=ORIENTED_EDGE('',*,*,#14235,.F.);
#18784=ORIENTED_EDGE('',*,*,#14251,.T.);
#18785=ORIENTED_EDGE('',*,*,#14236,.T.);
#18786=ORIENTED_EDGE('',*,*,#14237,.T.);
#18787=ORIENTED_EDGE('',*,*,#14251,.F.);
#18788=ORIENTED_EDGE('',*,*,#14252,.T.);
#18789=ORIENTED_EDGE('',*,*,#14253,.T.);
#18790=ORIENTED_EDGE('',*,*,#14254,.T.);
#18791=ORIENTED_EDGE('',*,*,#14255,.T.);
#18792=ORIENTED_EDGE('',*,*,#14256,.T.);
#18793=ORIENTED_EDGE('',*,*,#14257,.F.);
#18794=ORIENTED_EDGE('',*,*,#14256,.F.);
#18795=ORIENTED_EDGE('',*,*,#14254,.F.);
#18796=ORIENTED_EDGE('',*,*,#14253,.F.);
#18797=ORIENTED_EDGE('',*,*,#14252,.F.);
#18798=ORIENTED_EDGE('',*,*,#14258,.T.);
#18799=ORIENTED_EDGE('',*,*,#14259,.F.);
#18800=ORIENTED_EDGE('',*,*,#14260,.F.);
#18801=ORIENTED_EDGE('',*,*,#14261,.F.);
#18802=ORIENTED_EDGE('',*,*,#14262,.F.);
#18803=ORIENTED_EDGE('',*,*,#14263,.F.);
#18804=ORIENTED_EDGE('',*,*,#14264,.F.);
#18805=ORIENTED_EDGE('',*,*,#14265,.F.);
#18806=ORIENTED_EDGE('',*,*,#14266,.F.);
#18807=ORIENTED_EDGE('',*,*,#14267,.F.);
#18808=ORIENTED_EDGE('',*,*,#14268,.F.);
#18809=ORIENTED_EDGE('',*,*,#14269,.F.);
#18810=ORIENTED_EDGE('',*,*,#14270,.F.);
#18811=ORIENTED_EDGE('',*,*,#14271,.F.);
#18812=ORIENTED_EDGE('',*,*,#14258,.F.);
#18813=ORIENTED_EDGE('',*,*,#14271,.T.);
#18814=ORIENTED_EDGE('',*,*,#14272,.F.);
#18815=ORIENTED_EDGE('',*,*,#14273,.F.);
#18816=ORIENTED_EDGE('',*,*,#14269,.T.);
#18817=ORIENTED_EDGE('',*,*,#14274,.F.);
#18818=ORIENTED_EDGE('',*,*,#14275,.F.);
#18819=ORIENTED_EDGE('',*,*,#14267,.T.);
#18820=ORIENTED_EDGE('',*,*,#14276,.F.);
#18821=ORIENTED_EDGE('',*,*,#14277,.F.);
#18822=ORIENTED_EDGE('',*,*,#14265,.T.);
#18823=ORIENTED_EDGE('',*,*,#14278,.F.);
#18824=ORIENTED_EDGE('',*,*,#14279,.F.);
#18825=ORIENTED_EDGE('',*,*,#14263,.T.);
#18826=ORIENTED_EDGE('',*,*,#14280,.F.);
#18827=ORIENTED_EDGE('',*,*,#14281,.F.);
#18828=ORIENTED_EDGE('',*,*,#14261,.T.);
#18829=ORIENTED_EDGE('',*,*,#14282,.F.);
#18830=ORIENTED_EDGE('',*,*,#14283,.F.);
#18831=ORIENTED_EDGE('',*,*,#14259,.T.);
#18832=ORIENTED_EDGE('',*,*,#14250,.F.);
#18833=ORIENTED_EDGE('',*,*,#14284,.T.);
#18834=ORIENTED_EDGE('',*,*,#14277,.T.);
#18835=ORIENTED_EDGE('',*,*,#14276,.T.);
#18836=ORIENTED_EDGE('',*,*,#14266,.T.);
#18837=ORIENTED_EDGE('',*,*,#14284,.F.);
#18838=ORIENTED_EDGE('',*,*,#14249,.F.);
#18839=ORIENTED_EDGE('',*,*,#14285,.T.);
#18840=ORIENTED_EDGE('',*,*,#14279,.T.);
#18841=ORIENTED_EDGE('',*,*,#14278,.T.);
#18842=ORIENTED_EDGE('',*,*,#14264,.T.);
#18843=ORIENTED_EDGE('',*,*,#14285,.F.);
#18844=ORIENTED_EDGE('',*,*,#14245,.F.);
#18845=ORIENTED_EDGE('',*,*,#14286,.T.);
#18846=ORIENTED_EDGE('',*,*,#14281,.T.);
#18847=ORIENTED_EDGE('',*,*,#14280,.T.);
#18848=ORIENTED_EDGE('',*,*,#14262,.T.);
#18849=ORIENTED_EDGE('',*,*,#14286,.F.);
#18850=ORIENTED_EDGE('',*,*,#14244,.F.);
#18851=ORIENTED_EDGE('',*,*,#14241,.F.);
#18852=ORIENTED_EDGE('',*,*,#14248,.F.);
#18853=ORIENTED_EDGE('',*,*,#14287,.T.);
#18854=ORIENTED_EDGE('',*,*,#14283,.T.);
#18855=ORIENTED_EDGE('',*,*,#14282,.T.);
#18856=ORIENTED_EDGE('',*,*,#14260,.T.);
#18857=ORIENTED_EDGE('',*,*,#14287,.F.);
#18858=ORIENTED_EDGE('',*,*,#14247,.F.);
#18859=ORIENTED_EDGE('',*,*,#14288,.T.);
#18860=ORIENTED_EDGE('',*,*,#14273,.T.);
#18861=ORIENTED_EDGE('',*,*,#14272,.T.);
#18862=ORIENTED_EDGE('',*,*,#14270,.T.);
#18863=ORIENTED_EDGE('',*,*,#14288,.F.);
#18864=ORIENTED_EDGE('',*,*,#14246,.F.);
#18865=ORIENTED_EDGE('',*,*,#14289,.T.);
#18866=ORIENTED_EDGE('',*,*,#14275,.T.);
#18867=ORIENTED_EDGE('',*,*,#14274,.T.);
#18868=ORIENTED_EDGE('',*,*,#14268,.T.);
#18869=ORIENTED_EDGE('',*,*,#14289,.F.);
#18870=ORIENTED_EDGE('',*,*,#14257,.T.);
#18871=ORIENTED_EDGE('',*,*,#14290,.T.);
#18872=ORIENTED_EDGE('',*,*,#14291,.F.);
#18873=ORIENTED_EDGE('',*,*,#14290,.F.);
#18874=ORIENTED_EDGE('',*,*,#14292,.F.);
#18875=ORIENTED_EDGE('',*,*,#14291,.T.);
#18876=ORIENTED_EDGE('',*,*,#14243,.F.);
#18877=ORIENTED_EDGE('',*,*,#14293,.T.);
#18878=ORIENTED_EDGE('',*,*,#14292,.T.);
#18879=ORIENTED_EDGE('',*,*,#14293,.F.);
#18880=ORIENTED_EDGE('',*,*,#14294,.F.);
#18881=ORIENTED_EDGE('',*,*,#14295,.T.);
#18882=ORIENTED_EDGE('',*,*,#14239,.T.);
#18883=ORIENTED_EDGE('',*,*,#14295,.F.);
#18884=ORIENTED_EDGE('',*,*,#14294,.T.);
#18885=ORIENTED_EDGE('',*,*,#14296,.F.);
#18886=ORIENTED_EDGE('',*,*,#14296,.T.);
#18887=ORIENTED_EDGE('',*,*,#14297,.T.);
#18888=ORIENTED_EDGE('',*,*,#14255,.F.);
#18889=ORIENTED_EDGE('',*,*,#14297,.F.);
#25323=CONICAL_SURFACE('',#27422,3.0525,0.785398163397439);
#25324=CONICAL_SURFACE('',#27426,7.4,0.785398163397448);
#25325=CONICAL_SURFACE('',#27427,7.4,0.785398163397448);
#25326=CONICAL_SURFACE('',#27431,3.0525,0.785398163397448);
#25616=ADVANCED_FACE('',(#2803),#272,.T.);
#25617=ADVANCED_FACE('',(#2804),#597,.F.);
#25618=ADVANCED_FACE('',(#2805,#852,#853,#854,#855,#856,#857),#598,.T.);
#25619=ADVANCED_FACE('',(#2806),#273,.T.);
#25620=ADVANCED_FACE('',(#2807,#858),#599,.F.);
#25621=ADVANCED_FACE('',(#2808),#142,.T.);
#25622=ADVANCED_FACE('',(#2809),#600,.T.);
#25623=ADVANCED_FACE('',(#2810),#601,.T.);
#25624=ADVANCED_FACE('',(#2811),#602,.T.);
#25625=ADVANCED_FACE('',(#2812),#603,.T.);
#25626=ADVANCED_FACE('',(#2813),#604,.T.);
#25627=ADVANCED_FACE('',(#2814),#605,.T.);
#25628=ADVANCED_FACE('',(#2815),#25323,.F.);
#25629=ADVANCED_FACE('',(#2816,#859),#1763,.T.);
#25630=ADVANCED_FACE('',(#2817),#25324,.T.);
#25631=ADVANCED_FACE('',(#2818),#25325,.T.);
#25632=ADVANCED_FACE('',(#2819,#860),#1764,.T.);
#25633=ADVANCED_FACE('',(#2820),#25326,.F.);
#26876=CLOSED_SHELL('',(#25616,#25617,#25618,#25619,#25620,#25621,#25622,
#25623,#25624,#25625,#25626,#25627,#25628,#25629,#25630,#25631,#25632,#25633));
#27399=AXIS2_PLACEMENT_3D('',#44071,#29955,#29956);
#27400=AXIS2_PLACEMENT_3D('',#44465,#29958,#29959);
#27401=AXIS2_PLACEMENT_3D('',#44496,#29961,#29962);
#27402=AXIS2_PLACEMENT_3D('',#44498,#29963,#29964);
#27403=AXIS2_PLACEMENT_3D('',#44530,#29967,#29968);
#27404=AXIS2_PLACEMENT_3D('',#44942,#29970,#29971);
#27405=AXIS2_PLACEMENT_3D('',#44944,#29972,#29973);
#27406=AXIS2_PLACEMENT_3D('',#44947,#29975,#29976);
#27407=AXIS2_PLACEMENT_3D('',#44948,#29977,#29978);
#27408=AXIS2_PLACEMENT_3D('',#44950,#29979,#29980);
#27409=AXIS2_PLACEMENT_3D('',#44952,#29981,#29982);
#27410=AXIS2_PLACEMENT_3D('',#44981,#29983,#29984);
#27411=AXIS2_PLACEMENT_3D('',#45008,#29985,#29986);
#27412=AXIS2_PLACEMENT_3D('',#45037,#29987,#29988);
#27413=AXIS2_PLACEMENT_3D('',#45066,#29989,#29990);
#27414=AXIS2_PLACEMENT_3D('',#45093,#29991,#29992);
#27415=AXIS2_PLACEMENT_3D('',#45121,#29993,#29994);
#27416=AXIS2_PLACEMENT_3D('',#45312,#29995,#29996);
#27417=AXIS2_PLACEMENT_3D('',#45314,#29998,#29999);
#27418=AXIS2_PLACEMENT_3D('',#45316,#30001,#30002);
#27419=AXIS2_PLACEMENT_3D('',#45318,#30004,#30005);
#27420=AXIS2_PLACEMENT_3D('',#45320,#30007,#30008);
#27421=AXIS2_PLACEMENT_3D('',#45322,#30010,#30011);
#27422=AXIS2_PLACEMENT_3D('',#45324,#30013,#30014);
#27423=AXIS2_PLACEMENT_3D('',#45327,#30016,#30017);
#27424=AXIS2_PLACEMENT_3D('',#45328,#30018,#30019);
#27425=AXIS2_PLACEMENT_3D('',#45330,#30020,#30021);
#27426=AXIS2_PLACEMENT_3D('',#45331,#30022,#30023);
#27427=AXIS2_PLACEMENT_3D('',#45333,#30025,#30026);
#27428=AXIS2_PLACEMENT_3D('',#45335,#30027,#30028);
#27429=AXIS2_PLACEMENT_3D('',#45337,#30030,#30031);
#27430=AXIS2_PLACEMENT_3D('',#45339,#30032,#30033);
#27431=AXIS2_PLACEMENT_3D('',#45340,#30034,#30035);
#29955=DIRECTION('axis',(0.,0.,1.));
#29956=DIRECTION('refdir',(1.,0.,0.));
#29957=DIRECTION('',(0.747418957963599,8.91271585113921E-15,-0.664352994481554));
#29958=DIRECTION('center_axis',(0.,0.,1.));
#29959=DIRECTION('ref_axis',(1.,0.,0.));
#29960=DIRECTION('',(0.,0.,1.));
#29961=DIRECTION('center_axis',(0.,-1.,0.));
#29962=DIRECTION('ref_axis',(1.,0.,0.));
#29963=DIRECTION('center_axis',(0.,-1.,0.));
#29964=DIRECTION('ref_axis',(1.,0.,0.));
#29965=DIRECTION('',(0.,1.,0.));
#29966=DIRECTION('',(0.,1.,0.));
#29967=DIRECTION('center_axis',(0.,-1.,0.));
#29968=DIRECTION('ref_axis',(1.,0.,0.));
#29969=DIRECTION('',(0.000174853042027504,0.707106750910439,0.707106789843866));
#29970=DIRECTION('center_axis',(0.,-1.,0.));
#29971=DIRECTION('ref_axis',(1.,0.,0.));
#29972=DIRECTION('center_axis',(0.,-1.,0.));
#29973=DIRECTION('ref_axis',(1.,0.,0.));
#29974=DIRECTION('',(0.,1.,0.));
#29975=DIRECTION('center_axis',(0.,-1.,0.));
#29976=DIRECTION('ref_axis',(1.,0.,0.));
#29977=DIRECTION('center_axis',(0.,-1.,0.));
#29978=DIRECTION('ref_axis',(0.,0.,-1.));
#29979=DIRECTION('center_axis',(-1.,0.,-1.55820775385987E-16));
#29980=DIRECTION('ref_axis',(-1.55820775385987E-16,0.,1.));
#29981=DIRECTION('center_axis',(0.,1.,0.));
#29982=DIRECTION('ref_axis',(0.,0.,-1.));
#29983=DIRECTION('center_axis',(0.,1.,0.));
#29984=DIRECTION('ref_axis',(0.,0.,-1.));
#29985=DIRECTION('center_axis',(0.,1.,0.));
#29986=DIRECTION('ref_axis',(0.,0.,-1.));
#29987=DIRECTION('center_axis',(0.,1.,0.));
#29988=DIRECTION('ref_axis',(0.,0.,-1.));
#29989=DIRECTION('center_axis',(0.,1.,0.));
#29990=DIRECTION('ref_axis',(0.,0.,-1.));
#29991=DIRECTION('center_axis',(0.,1.,0.));
#29992=DIRECTION('ref_axis',(0.,0.,-1.));
#29993=DIRECTION('center_axis',(0.,1.,0.));
#29994=DIRECTION('ref_axis',(0.,0.,-1.));
#29995=DIRECTION('center_axis',(-0.500000000000001,0.,0.866025403784438));
#29996=DIRECTION('ref_axis',(0.866025403784439,0.,0.499999999999999));
#29997=DIRECTION('',(0.500000000000001,0.,-0.866025403784438));
#29998=DIRECTION('center_axis',(0.500000000000001,0.,0.866025403784438));
#29999=DIRECTION('ref_axis',(0.866025403784437,0.,-0.500000000000002));
#30000=DIRECTION('',(-0.500000000000001,0.,-0.866025403784438));
#30001=DIRECTION('center_axis',(1.,0.,0.));
#30002=DIRECTION('ref_axis',(0.,0.,-1.));
#30003=DIRECTION('',(-1.,0.,0.));
#30004=DIRECTION('center_axis',(0.5,0.,-0.866025403784439));
#30005=DIRECTION('ref_axis',(-0.866025403784439,0.,-0.5));
#30006=DIRECTION('',(-0.5,0.,0.866025403784439));
#30007=DIRECTION('center_axis',(-0.500000000000001,0.,-0.866025403784438));
#30008=DIRECTION('ref_axis',(-0.866025403784437,0.,0.500000000000003));
#30009=DIRECTION('',(0.500000000000001,0.,0.866025403784438));
#30010=DIRECTION('center_axis',(-1.,0.,0.));
#30011=DIRECTION('ref_axis',(0.,0.,1.));
#30012=DIRECTION('',(1.,0.,0.));
#30013=DIRECTION('center_axis',(0.,1.,0.));
#30014=DIRECTION('ref_axis',(1.,0.,0.));
#30015=DIRECTION('',(-0.707106781186541,0.707106781186554,-8.65956056235486E-17));
#30016=DIRECTION('center_axis',(0.,-1.,0.));
#30017=DIRECTION('ref_axis',(1.,0.,0.));
#30018=DIRECTION('center_axis',(0.,1.,0.));
#30019=DIRECTION('ref_axis',(0.,0.,1.));
#30020=DIRECTION('center_axis',(0.,-1.,0.));
#30021=DIRECTION('ref_axis',(1.,0.,0.));
#30022=DIRECTION('center_axis',(0.,-1.,0.));
#30023=DIRECTION('ref_axis',(1.,0.,0.));
#30024=DIRECTION('',(0.707106781186548,0.707106781186548,8.65956056235493E-17));
#30025=DIRECTION('center_axis',(0.,1.,0.));
#30026=DIRECTION('ref_axis',(1.,0.,0.));
#30027=DIRECTION('center_axis',(0.,-1.,0.));
#30028=DIRECTION('ref_axis',(1.,0.,0.));
#30029=DIRECTION('',(-0.707106781186548,0.707106781186548,-8.65956056235493E-17));
#30030=DIRECTION('center_axis',(0.,-1.,0.));
#30031=DIRECTION('ref_axis',(0.,0.,-1.));
#30032=DIRECTION('center_axis',(0.,-1.,0.));
#30033=DIRECTION('ref_axis',(1.,0.,0.));
#30034=DIRECTION('center_axis',(0.,-1.,0.));
#30035=DIRECTION('ref_axis',(1.,0.,0.));
#30036=DIRECTION('',(0.707106781186547,0.707106781186547,8.65956056235493E-17));
#44071=CARTESIAN_POINT('',(0.,0.,0.));
#44072=CARTESIAN_POINT('Ctrl Pts',(8.35603499314338,15.8,85.4390826561945));
#44073=CARTESIAN_POINT('Ctrl Pts',(8.35603499314338,15.9372797480275,85.4390826561945));
#44074=CARTESIAN_POINT('Ctrl Pts',(8.39668257439119,16.1218710106354,85.4444904181629));
#44075=CARTESIAN_POINT('Ctrl Pts',(8.48962600103117,16.2884083933886,85.4549757803719));
#44076=CARTESIAN_POINT('Ctrl Pts',(8.51904255235788,16.333616011952,85.4581256707728));
#44077=CARTESIAN_POINT('Ctrl Pts',(8.53434287032992,16.3557032208687,85.4597347029858));
#44078=CARTESIAN_POINT('Ctrl Pts',(8.55014120211907,16.3772240255913,85.4613625335412));
#44079=CARTESIAN_POINT('Ctrl Pts',(8.60474859865648,16.4472645215626,85.4668665636608));
#44080=CARTESIAN_POINT('Ctrl Pts',(8.66423709283022,16.5065301286674,85.472314639594));
#44081=CARTESIAN_POINT('Ctrl Pts',(8.73421571262732,16.5611896429675,85.477810600089));
#44082=CARTESIAN_POINT('Ctrl Pts',(8.76289021098275,16.5822842616593,85.4799785377766));
#44083=CARTESIAN_POINT('Ctrl Pts',(8.80015375962284,16.6073660501337,85.4826344158676));
#44084=CARTESIAN_POINT('Ctrl Pts',(8.84680287582055,16.6350364303463,85.4856715584966));
#44085=CARTESIAN_POINT('Ctrl Pts',(8.91126359072523,16.6684953457075,85.489460606674));
#44086=CARTESIAN_POINT('Ctrl Pts',(8.97879268762966,16.6964087072018,85.4927632839475));
#44087=CARTESIAN_POINT('Ctrl Pts',(9.04794555696647,16.7183902183462,85.4954326308204));
#44088=CARTESIAN_POINT('Ctrl Pts',(9.22435588573701,16.7630993137503,85.5009743602204));
#44089=CARTESIAN_POINT('Ctrl Pts',(9.37978678214075,16.7631990287376,85.5009941213014));
#44090=CARTESIAN_POINT('Ctrl Pts',(9.52362841368894,16.7304680703605,85.4969281164271));
#44091=CARTESIAN_POINT('Ctrl Pts',(9.52948187007311,16.7291027348195,85.4967587924218));
#44092=CARTESIAN_POINT('Ctrl Pts',(9.53972603545934,16.7266396251387,85.4964537623072));
#44093=CARTESIAN_POINT('Ctrl Pts',(9.55140693128475,16.7236542968834,85.4960853644285));
#44094=CARTESIAN_POINT('Ctrl Pts',(9.56305629792811,16.7204997032745,85.4956975301883));
#44095=CARTESIAN_POINT('Ctrl Pts',(9.5746828868594,16.7172323247418,85.4952968805524));
#44096=CARTESIAN_POINT('Ctrl Pts',(9.6065596797669,16.7077838948382,85.4941429373237));
#44097=CARTESIAN_POINT('Ctrl Pts',(9.65813475370038,16.6898037484486,85.4919764613753));
#44098=CARTESIAN_POINT('Ctrl Pts',(9.72483636139708,16.6606586538393,85.4885662989555));
#44099=CARTESIAN_POINT('Ctrl Pts',(9.81035193883595,16.6152393568737,85.4834442118835));
#44100=CARTESIAN_POINT('Ctrl Pts',(9.88952955214136,16.5608297157303,85.477681416797));
#44101=CARTESIAN_POINT('Ctrl Pts',(9.96015984107354,16.4995598748089,85.4717656307727));
#44102=CARTESIAN_POINT('Ctrl Pts',(10.0566824559075,16.4030718438372,85.4630358281122));
#44103=CARTESIAN_POINT('Ctrl Pts',(10.140445547261,16.2824959491676,85.4539873067033));
#44104=CARTESIAN_POINT('Ctrl Pts',(10.1985441116753,16.1489861273042,85.4471485778523));
#44105=CARTESIAN_POINT('Ctrl Pts',(10.222497181123,16.0801829715165,85.4442465721495));
#44106=CARTESIAN_POINT('Ctrl Pts',(10.2411110001271,16.0101477612633,85.441938174718));
#44107=CARTESIAN_POINT('Ctrl Pts',(10.2671411860703,15.8682847284844,85.4386400439914));
#44108=CARTESIAN_POINT('Ctrl Pts',(10.2676702177296,15.7087996732268,85.4385975861224));
#44109=CARTESIAN_POINT('Ctrl Pts',(10.2253511275564,15.5187131618124,85.4439361201402));
#44110=CARTESIAN_POINT('Ctrl Pts',(10.1635097686491,15.3605723341138,85.4513910623746));
#44111=CARTESIAN_POINT('Ctrl Pts',(10.0582364282556,15.1952877308291,85.4629318702328));
#44112=CARTESIAN_POINT('Ctrl Pts',(9.93758658799873,15.0752327539855,85.4740118542376));
#44113=CARTESIAN_POINT('Ctrl Pts',(9.82095295951565,14.9912740599348,85.4827275167418));
#44114=CARTESIAN_POINT('Ctrl Pts',(9.7257726708022,14.938502416334,85.48864489927));
#44115=CARTESIAN_POINT('Ctrl Pts',(9.64154714023013,14.9035142378301,85.4927752312384));
#44116=CARTESIAN_POINT('Ctrl Pts',(9.58527096084076,14.8856853198025,85.4949434208681));
#44117=CARTESIAN_POINT('Ctrl Pts',(9.55910119355026,14.8783947067353,85.4958378446216));
#44118=CARTESIAN_POINT('Ctrl Pts',(9.54597200279266,14.8749411777993,85.4962632794556));
#44119=CARTESIAN_POINT('Ctrl Pts',(9.53283457660932,14.8716784688763,85.4966665696332));
#44120=CARTESIAN_POINT('Ctrl Pts',(9.45354917166566,14.8532449033689,85.4989535397092));
#44121=CARTESIAN_POINT('Ctrl Pts',(9.31002212387416,14.8376927917007,85.5009593430419));
#44122=CARTESIAN_POINT('Ctrl Pts',(9.15304234143535,14.8547157047969,85.4987606437473));
#44123=CARTESIAN_POINT('Ctrl Pts',(9.04735019561901,14.8816229494821,85.4954334077506));
#44124=CARTESIAN_POINT('Ctrl Pts',(8.97819116088274,14.903593487749,85.4927637202553));
#44125=CARTESIAN_POINT('Ctrl Pts',(8.89391110377091,14.9384727132614,85.4886374013684));
#44126=CARTESIAN_POINT('Ctrl Pts',(8.81450469736164,14.9826783322091,85.4836911519947));
#44127=CARTESIAN_POINT('Ctrl Pts',(8.75499655724527,15.0226900205634,85.4794515057453));
#44128=CARTESIAN_POINT('Ctrl Pts',(8.66971693517491,15.0875063099098,85.4728628549599));
#44129=CARTESIAN_POINT('Ctrl Pts',(8.60739958396077,15.1498071578507,85.4671368089765));
#44130=CARTESIAN_POINT('Ctrl Pts',(8.55799266459696,15.2123260535644,85.4621833875471));
#44131=CARTESIAN_POINT('Ctrl Pts',(8.54720257389172,15.2263954689324,85.4610892717717));
#44132=CARTESIAN_POINT('Ctrl Pts',(8.52873347530619,15.2515214314165,85.4591853935954));
#44133=CARTESIAN_POINT('Ctrl Pts',(8.49372813179311,15.3037099876317,85.4554712250094));
#44134=CARTESIAN_POINT('Ctrl Pts',(8.39640281859525,15.4781780558787,85.4444905178981));
#44135=CARTESIAN_POINT('Ctrl Pts',(8.35603499314338,15.6627202519725,85.4390826561945));
#44136=CARTESIAN_POINT('Ctrl Pts',(8.35603499314338,15.8,85.4390826561945));
#44137=CARTESIAN_POINT('Ctrl Pts',(8.40568999542892,15.8,85.3949461660668));
#44138=CARTESIAN_POINT('Ctrl Pts',(8.40568999542892,15.9308326910989,85.3949461660668));
#44139=CARTESIAN_POINT('Ctrl Pts',(8.44474272963522,16.1067243580164,85.3998613101596));
#44140=CARTESIAN_POINT('Ctrl Pts',(8.53356913858795,16.2648067705402,85.4093648382305));
#44141=CARTESIAN_POINT('Ctrl Pts',(8.56164483771783,16.3076765997574,85.4122177047785));
#44142=CARTESIAN_POINT('Ctrl Pts',(8.57624129470615,16.3286119068441,85.4136746517426));
#44143=CARTESIAN_POINT('Ctrl Pts',(8.59130554481547,16.349001315578,85.4151482154668));
#44144=CARTESIAN_POINT('Ctrl Pts',(8.64334979487582,16.4153281666897,85.420129275667));
#44145=CARTESIAN_POINT('Ctrl Pts',(8.69993120799356,16.4713215409808,85.4250535045443));
#44146=CARTESIAN_POINT('Ctrl Pts',(8.76632846975484,16.5228636831985,85.4300144910158));
#44147=CARTESIAN_POINT('Ctrl Pts',(8.79352158354697,16.5427454911753,85.4319708237179));
#44148=CARTESIAN_POINT('Ctrl Pts',(8.82883414057959,16.5663683097786,85.4343664168167));
#44149=CARTESIAN_POINT('Ctrl Pts',(8.87299808292085,16.5924050133844,85.4371043307198));
#44150=CARTESIAN_POINT('Ctrl Pts',(8.93396931795387,16.6238611980788,85.4405182224936));
#44151=CARTESIAN_POINT('Ctrl Pts',(8.9977612650961,16.650069132683,85.4434914376289));
#44152=CARTESIAN_POINT('Ctrl Pts',(9.06301962035174,16.6706899553159,85.4458931740141));
#44153=CARTESIAN_POINT('Ctrl Pts',(9.22939703062867,16.7126018503172,85.450877074459));
#44154=CARTESIAN_POINT('Ctrl Pts',(9.37567654308211,16.7126937732917,85.450894746136));
#44155=CARTESIAN_POINT('Ctrl Pts',(9.5113086780914,16.6820130652668,85.447238215881));
#44156=CARTESIAN_POINT('Ctrl Pts',(9.51682828834093,16.6807331755622,85.4470859379221));
#44157=CARTESIAN_POINT('Ctrl Pts',(9.52648877180839,16.6784240983265,85.4468116069232));
#44158=CARTESIAN_POINT('Ctrl Pts',(9.53750552568468,16.6756251154288,85.4464802597071));
#44159=CARTESIAN_POINT('Ctrl Pts',(9.5484940380417,16.6726670462954,85.4461314016811));
#44160=CARTESIAN_POINT('Ctrl Pts',(9.55946209396692,16.6696029422388,85.4457709954931));
#44161=CARTESIAN_POINT('Ctrl Pts',(9.58953773286542,16.6607411172119,85.4447328699376));
#44162=CARTESIAN_POINT('Ctrl Pts',(9.63822376367679,16.6438696842517,85.4427832798092));
#44163=CARTESIAN_POINT('Ctrl Pts',(9.70125198646232,16.6164958184463,85.4397126409855));
#44164=CARTESIAN_POINT('Ctrl Pts',(9.7821498111748,16.5737901734561,85.435097370155));
#44165=CARTESIAN_POINT('Ctrl Pts',(9.85719664323122,16.5225446594837,85.4298991149593));
#44166=CARTESIAN_POINT('Ctrl Pts',(9.92427648325852,16.4647182760809,85.4245561933527));
#44167=CARTESIAN_POINT('Ctrl Pts',(10.0160651871645,16.3735429235342,85.4166660324392));
#44168=CARTESIAN_POINT('Ctrl Pts',(10.0960218795394,16.2592652524798,85.4084709487996));
#44169=CARTESIAN_POINT('Ctrl Pts',(10.1516154183529,16.1323600396269,85.4022682199982));
#44170=CARTESIAN_POINT('Ctrl Pts',(10.174555475083,16.0669058752731,85.3996349002206));
#44171=CARTESIAN_POINT('Ctrl Pts',(10.1923954028737,16.0002310501117,85.3975393727227));
#44172=CARTESIAN_POINT('Ctrl Pts',(10.2173610140913,15.8651024456785,85.3945442463104));
#44173=CARTESIAN_POINT('Ctrl Pts',(10.21786262709,15.7130489813637,85.3945060111475));
#44174=CARTESIAN_POINT('Ctrl Pts',(10.1772803096206,15.5320202482537,85.3993536913281));
#44175=CARTESIAN_POINT('Ctrl Pts',(10.1180642105147,15.3816292809796,85.4061177055654));
#44176=CARTESIAN_POINT('Ctrl Pts',(10.0175327140903,15.2248716877216,85.4165730172062));
#44177=CARTESIAN_POINT('Ctrl Pts',(9.90277676210439,15.1114513230244,85.4265874895966));
#44178=CARTESIAN_POINT('Ctrl Pts',(9.79218928037887,15.0323392040438,85.4344512288155));
#44179=CARTESIAN_POINT('Ctrl Pts',(9.7021216365312,14.982710988249,85.4397838923364));
#44180=CARTESIAN_POINT('Ctrl Pts',(9.62255624266952,14.9498587840303,85.4435022587664));
#44181=CARTESIAN_POINT('Ctrl Pts',(9.5694496368992,14.9331342462661,85.4454530300753));
#44182=CARTESIAN_POINT('Ctrl Pts',(9.54476270274329,14.9262973372286,85.4462576016557));
#44183=CARTESIAN_POINT('Ctrl Pts',(9.53237917313348,14.9230591782846,85.4466402647976));
#44184=CARTESIAN_POINT('Ctrl Pts',(9.51998948264082,14.9200003032379,85.4470029819006));
#44185=CARTESIAN_POINT('Ctrl Pts',(9.44522624547653,14.9027206181603,85.4490596970557));
#44186=CARTESIAN_POINT('Ctrl Pts',(9.31001995354237,14.888162924871,85.4508618929458));
#44187=CARTESIAN_POINT('Ctrl Pts',(9.16214069815493,14.9040969243232,85.4488863553164));
#44188=CARTESIAN_POINT('Ctrl Pts',(9.06245933788975,14.9293229082359,85.4458938636106));
#44189=CARTESIAN_POINT('Ctrl Pts',(8.9971950546273,14.9499329681114,85.4434918584837));
#44190=CARTESIAN_POINT('Ctrl Pts',(8.9175790894704,14.9826813768387,85.4397771417074));
#44191=CARTESIAN_POINT('Ctrl Pts',(8.84243666780698,15.0242555638747,85.4353195904802));
#44192=CARTESIAN_POINT('Ctrl Pts',(8.78604443295927,15.0619394025398,85.431495454472));
#44193=CARTESIAN_POINT('Ctrl Pts',(8.70514823333775,15.1230441827598,85.4255490150097));
#44194=CARTESIAN_POINT('Ctrl Pts',(8.64587417668115,15.1819052888515,85.4203735430612));
#44195=CARTESIAN_POINT('Ctrl Pts',(8.59879194533658,15.2411027726911,85.4158910836619));
#44196=CARTESIAN_POINT('Ctrl Pts',(8.58850699900074,15.2544279222765,85.4149008595262));
#44197=CARTESIAN_POINT('Ctrl Pts',(8.57089587702538,15.2782326333794,85.4131773950912));
#44198=CARTESIAN_POINT('Ctrl Pts',(8.53749381124016,15.3277115849179,85.4098139059006));
#44199=CARTESIAN_POINT('Ctrl Pts',(8.44447962066645,15.4933224411837,85.3998614319814));
#44200=CARTESIAN_POINT('Ctrl Pts',(8.40568999542892,15.6691673089011,85.3949461660668));
#44201=CARTESIAN_POINT('Ctrl Pts',(8.40568999542892,15.8,85.3949461660668));
#44202=CARTESIAN_POINT('Ctrl Pts',(8.45534499771446,15.8,85.3508096759391));
#44203=CARTESIAN_POINT('Ctrl Pts',(8.45534499771446,15.9243856341704,85.3508096759391));
#44204=CARTESIAN_POINT('Ctrl Pts',(8.49280288487924,16.0915777053974,85.3552322021562));
#44205=CARTESIAN_POINT('Ctrl Pts',(8.57751227614473,16.2412051476919,85.3637538960892));
#44206=CARTESIAN_POINT('Ctrl Pts',(8.60424712307778,16.2817371875628,85.3663097387841));
#44207=CARTESIAN_POINT('Ctrl Pts',(8.61813971908238,16.3015205928195,85.3676146004995));
#44208=CARTESIAN_POINT('Ctrl Pts',(8.63246988751186,16.3207786055647,85.3689338973923));
#44209=CARTESIAN_POINT('Ctrl Pts',(8.68195099109516,16.3833918118167,85.3733919876731));
#44210=CARTESIAN_POINT('Ctrl Pts',(8.7356253231569,16.4361129532943,85.3777923694946));
#44211=CARTESIAN_POINT('Ctrl Pts',(8.79844122688236,16.4845377234294,85.3822183819425));
#44212=CARTESIAN_POINT('Ctrl Pts',(8.82415295611118,16.5032067206913,85.3839631096591));
#44213=CARTESIAN_POINT('Ctrl Pts',(8.85751452153635,16.5253705694234,85.3860984177658));
#44214=CARTESIAN_POINT('Ctrl Pts',(8.89919329002115,16.5497735964226,85.3885371029431));
#44215=CARTESIAN_POINT('Ctrl Pts',(8.95667504518251,16.5792270504501,85.3915758383132));
#44216=CARTESIAN_POINT('Ctrl Pts',(9.01672984256254,16.6037295581642,85.3942195913102));
#44217=CARTESIAN_POINT('Ctrl Pts',(9.07809368373701,16.6229896922856,85.3963537172078));
#44218=CARTESIAN_POINT('Ctrl Pts',(9.23443817552033,16.6621043868841,85.4007797886977));
#44219=CARTESIAN_POINT('Ctrl Pts',(9.37156630402344,16.6621885178458,85.4007953709705));
#44220=CARTESIAN_POINT('Ctrl Pts',(9.49898894249385,16.633558060173,85.397548315335));
#44221=CARTESIAN_POINT('Ctrl Pts',(9.50417470660875,16.6323636163049,85.3974130834225));
#44222=CARTESIAN_POINT('Ctrl Pts',(9.51325150815744,16.6302085715143,85.3971694515393));
#44223=CARTESIAN_POINT('Ctrl Pts',(9.5236041200846,16.6275959339742,85.3968751549858));
#44224=CARTESIAN_POINT('Ctrl Pts',(9.53393177815528,16.6248343893163,85.3965652731739));
#44225=CARTESIAN_POINT('Ctrl Pts',(9.54424130107443,16.6219735597358,85.3962451104339));
#44226=CARTESIAN_POINT('Ctrl Pts',(9.57251578596394,16.6136983395856,85.3953228025516));
#44227=CARTESIAN_POINT('Ctrl Pts',(9.61831277365319,16.5979356200548,85.3935900982431));
#44228=CARTESIAN_POINT('Ctrl Pts',(9.67766761152756,16.5723329830534,85.3908589830154));
#44229=CARTESIAN_POINT('Ctrl Pts',(9.75394768351365,16.5323409900384,85.3867505284264));
#44230=CARTESIAN_POINT('Ctrl Pts',(9.82486373432107,16.4842596032372,85.3821168131216));
#44231=CARTESIAN_POINT('Ctrl Pts',(9.8883931254435,16.4298766773529,85.3773467559326));
#44232=CARTESIAN_POINT('Ctrl Pts',(9.97544791842136,16.3440140032313,85.3702962367661));
#44233=CARTESIAN_POINT('Ctrl Pts',(10.0515982118178,16.236034555792,85.362954590896));
#44234=CARTESIAN_POINT('Ctrl Pts',(10.1046867250305,16.1157339519497,85.3573878621441));
#44235=CARTESIAN_POINT('Ctrl Pts',(10.126613769043,16.0536287790298,85.3550232282919));
#44236=CARTESIAN_POINT('Ctrl Pts',(10.1436798056203,15.9903143389601,85.3531405707274));
#44237=CARTESIAN_POINT('Ctrl Pts',(10.1675808421122,15.8619201628725,85.3504484486294));
#44238=CARTESIAN_POINT('Ctrl Pts',(10.1680550364504,15.7172982895006,85.3504144361727));
#44239=CARTESIAN_POINT('Ctrl Pts',(10.1292094916849,15.5453273346951,85.3547712625161));
#44240=CARTESIAN_POINT('Ctrl Pts',(10.0726186523802,15.4026862278453,85.3608443487561));
#44241=CARTESIAN_POINT('Ctrl Pts',(9.97682899992489,15.2544556446141,85.3702141641797));
#44242=CARTESIAN_POINT('Ctrl Pts',(9.86796693621007,15.1476698920632,85.3791631249556));
#44243=CARTESIAN_POINT('Ctrl Pts',(9.76342560124209,15.0734043481528,85.3861749408892));
#44244=CARTESIAN_POINT('Ctrl Pts',(9.6784706022602,15.026919560164,85.3909228854027));
#44245=CARTESIAN_POINT('Ctrl Pts',(9.60356534510891,14.9962033302305,85.3942292862944));
#44246=CARTESIAN_POINT('Ctrl Pts',(9.55362831295764,14.9805831727297,85.3959626392824));
#44247=CARTESIAN_POINT('Ctrl Pts',(9.53042421193632,14.974199967722,85.3966773586898));
#44248=CARTESIAN_POINT('Ctrl Pts',(9.5187863434743,14.97117717877,85.3970172501395));
#44249=CARTESIAN_POINT('Ctrl Pts',(9.50714438867232,14.9683221375996,85.3973393941678));
#44250=CARTESIAN_POINT('Ctrl Pts',(9.43690331928739,14.9521963329518,85.3991658544022));
#44251=CARTESIAN_POINT('Ctrl Pts',(9.31001778321058,14.9386330580413,85.4007644428496));
#44252=CARTESIAN_POINT('Ctrl Pts',(9.17123905487452,14.9534781438495,85.3990120668856));
#44253=CARTESIAN_POINT('Ctrl Pts',(9.07756848016049,14.9770228669897,85.3963543194706));
#44254=CARTESIAN_POINT('Ctrl Pts',(9.01619894837186,14.9962724484738,85.394219996712));
#44255=CARTESIAN_POINT('Ctrl Pts',(8.9412470751699,15.026890040416,85.3909168820463));
#44256=CARTESIAN_POINT('Ctrl Pts',(8.87036863825231,15.0658327955402,85.3869480289657));
#44257=CARTESIAN_POINT('Ctrl Pts',(8.81709230867327,15.1011887845163,85.3835394031987));
#44258=CARTESIAN_POINT('Ctrl Pts',(8.74057953150059,15.1585820556098,85.3782351750594));
#44259=CARTESIAN_POINT('Ctrl Pts',(8.68434876940152,15.2140034198523,85.3736102771458));
#44260=CARTESIAN_POINT('Ctrl Pts',(8.63959122607621,15.2698794918178,85.3695987797766));
#44261=CARTESIAN_POINT('Ctrl Pts',(8.62981142410976,15.2824603756206,85.3687124472807));
#44262=CARTESIAN_POINT('Ctrl Pts',(8.61305827874456,15.3049438353424,85.367169396587));
#44263=CARTESIAN_POINT('Ctrl Pts',(8.58125949068721,15.3517131822041,85.3641565867918));
#44264=CARTESIAN_POINT('Ctrl Pts',(8.49255642273764,15.5084668264888,85.3552323460647));
#44265=CARTESIAN_POINT('Ctrl Pts',(8.45534499771446,15.6756143658296,85.3508096759391));
#44266=CARTESIAN_POINT('Ctrl Pts',(8.45534499771446,15.8,85.3508096759391));
#44267=CARTESIAN_POINT('Ctrl Pts',(8.505,15.8,85.3066731858115));
#44268=CARTESIAN_POINT('Ctrl Pts',(8.505,15.9179385772418,85.3066731858115));
#44269=CARTESIAN_POINT('Ctrl Pts',(8.54086304012327,16.0764310527784,85.3106030941529));
#44270=CARTESIAN_POINT('Ctrl Pts',(8.62145541370151,16.2176035248435,85.3181429539479));
#44271=CARTESIAN_POINT('Ctrl Pts',(8.64684940843773,16.2557977753682,85.3204017727898));
#44272=CARTESIAN_POINT('Ctrl Pts',(8.66003814345861,16.2744292787949,85.3215545492563));
#44273=CARTESIAN_POINT('Ctrl Pts',(8.67363423020825,16.2925558955514,85.3227195793178));
#44274=CARTESIAN_POINT('Ctrl Pts',(8.7205521873145,16.3514554569438,85.3266546996792));
#44275=CARTESIAN_POINT('Ctrl Pts',(8.77131943832023,16.4009043656078,85.3305312344449));
#44276=CARTESIAN_POINT('Ctrl Pts',(8.83055398400987,16.4462117636603,85.3344222728693));
#44277=CARTESIAN_POINT('Ctrl Pts',(8.8547843286754,16.4636679502074,85.3359553956004));
#44278=CARTESIAN_POINT('Ctrl Pts',(8.8861949024931,16.4843728290683,85.3378304187148));
#44279=CARTESIAN_POINT('Ctrl Pts',(8.92538849712145,16.5071421794607,85.3399698751664));
#44280=CARTESIAN_POINT('Ctrl Pts',(8.97938077241115,16.5345929028214,85.3426334541328));
#44281=CARTESIAN_POINT('Ctrl Pts',(9.03569842002898,16.5573899836454,85.3449477449916));
#44282=CARTESIAN_POINT('Ctrl Pts',(9.09316774712228,16.5752894292553,85.3468142604014));
#44283=CARTESIAN_POINT('Ctrl Pts',(9.23947932041198,16.611606923451,85.3506825029363));
#44284=CARTESIAN_POINT('Ctrl Pts',(9.36745606496479,16.6116832623999,85.3506959958052));
#44285=CARTESIAN_POINT('Ctrl Pts',(9.4866692068963,16.5851030550793,85.3478584147889));
#44286=CARTESIAN_POINT('Ctrl Pts',(9.49152112487657,16.5839940570477,85.3477402289228));
#44287=CARTESIAN_POINT('Ctrl Pts',(9.50001424450649,16.581993044702,85.3475272961553));
#44288=CARTESIAN_POINT('Ctrl Pts',(9.50970271448452,16.5795667525196,85.3472700502645));
#44289=CARTESIAN_POINT('Ctrl Pts',(9.51936951826886,16.5770017323372,85.3469991446667));
#44290=CARTESIAN_POINT('Ctrl Pts',(9.52902050818195,16.5743441772328,85.3467192253746));
#44291=CARTESIAN_POINT('Ctrl Pts',(9.55549383906246,16.5666555619593,85.3459127351656));
#44292=CARTESIAN_POINT('Ctrl Pts',(9.59840178362959,16.5520015558579,85.344396916677));
#44293=CARTESIAN_POINT('Ctrl Pts',(9.6540832365928,16.5281701476604,85.3420053250454));
#44294=CARTESIAN_POINT('Ctrl Pts',(9.72574555585249,16.4908918066207,85.3384036866979));
#44295=CARTESIAN_POINT('Ctrl Pts',(9.79253082541093,16.4459745469907,85.3343345112839));
#44296=CARTESIAN_POINT('Ctrl Pts',(9.85250976762847,16.3950350786248,85.3301373185125));
#44297=CARTESIAN_POINT('Ctrl Pts',(9.93483064967827,16.3144850829283,85.3239264410931));
#44298=CARTESIAN_POINT('Ctrl Pts',(10.0071745440962,16.2128038591041,85.3174382329924));
#44299=CARTESIAN_POINT('Ctrl Pts',(10.057758031708,16.0991078642724,85.3125075042899));
#44300=CARTESIAN_POINT('Ctrl Pts',(10.078672063003,16.0403516827864,85.3104115563631));
#44301=CARTESIAN_POINT('Ctrl Pts',(10.0949642083669,15.9803976278085,85.3087417687321));
#44302=CARTESIAN_POINT('Ctrl Pts',(10.1178006701332,15.8587378800666,85.3063526509483));
#44303=CARTESIAN_POINT('Ctrl Pts',(10.1182474458107,15.7215475976374,85.3063228611977));
#44304=CARTESIAN_POINT('Ctrl Pts',(10.0811386737492,15.5586344211364,85.310188833704));
#44305=CARTESIAN_POINT('Ctrl Pts',(10.0271730942457,15.4237431747111,85.3155709919468));
#44306=CARTESIAN_POINT('Ctrl Pts',(9.93612528575951,15.2840396015067,85.3238553111532));
#44307=CARTESIAN_POINT('Ctrl Pts',(9.83315711031573,15.1838884611021,85.3317387603146));
#44308=CARTESIAN_POINT('Ctrl Pts',(9.7346619221053,15.1144694922618,85.3378986529629));
#44309=CARTESIAN_POINT('Ctrl Pts',(9.6548195679892,15.0711281320789,85.342061878469));
#44310=CARTESIAN_POINT('Ctrl Pts',(9.5845744475483,15.0425478764307,85.3449563138224));
#44311=CARTESIAN_POINT('Ctrl Pts',(9.53780698901607,15.0280320991933,85.3464722484895));
#44312=CARTESIAN_POINT('Ctrl Pts',(9.51608572112935,15.0221025982153,85.3470971157239));
#44313=CARTESIAN_POINT('Ctrl Pts',(9.50519351381511,15.0192951792553,85.3473942354814));
#44314=CARTESIAN_POINT('Ctrl Pts',(9.49429929470381,15.0166439719612,85.3476758064351));
#44315=CARTESIAN_POINT('Ctrl Pts',(9.42858039309825,15.0016720477432,85.3492720117487));
#44316=CARTESIAN_POINT('Ctrl Pts',(9.31001561287879,14.9891031912116,85.3506669927535));
#44317=CARTESIAN_POINT('Ctrl Pts',(9.1803374115941,15.0028593633758,85.3491377784547));
#44318=CARTESIAN_POINT('Ctrl Pts',(9.09267762243124,15.0247228257435,85.3468147753307));
#44319=CARTESIAN_POINT('Ctrl Pts',(9.03520284211642,15.0426119288362,85.3449481349403));
#44320=CARTESIAN_POINT('Ctrl Pts',(8.96491506086939,15.0710987039933,85.3420566223853));
#44321=CARTESIAN_POINT('Ctrl Pts',(8.89830060869765,15.1074100272057,85.3385764674512));
#44322=CARTESIAN_POINT('Ctrl Pts',(8.84814018438728,15.1404381664927,85.3355833519254));
#44323=CARTESIAN_POINT('Ctrl Pts',(8.77601082966343,15.1941199284598,85.3309213351092));
#44324=CARTESIAN_POINT('Ctrl Pts',(8.7228233621219,15.246101550853,85.3268470112305));
#44325=CARTESIAN_POINT('Ctrl Pts',(8.68039050681583,15.2986562109445,85.3233064758915));
#44326=CARTESIAN_POINT('Ctrl Pts',(8.67111584921878,15.3104928289646,85.3225240350353));
#44327=CARTESIAN_POINT('Ctrl Pts',(8.65522068046374,15.3316550373053,85.3211613980828));
#44328=CARTESIAN_POINT('Ctrl Pts',(8.62502517013426,15.3757147794904,85.3184992676831));
#44329=CARTESIAN_POINT('Ctrl Pts',(8.54063322480884,15.5236112117938,85.310603260148));
#44330=CARTESIAN_POINT('Ctrl Pts',(8.505,15.6820614227582,85.3066731858115));
#44331=CARTESIAN_POINT('Ctrl Pts',(8.505,15.8,85.3066731858115));
#44332=CARTESIAN_POINT('',(8.35603499314338,15.8,85.4390826561945));
#44333=CARTESIAN_POINT('',(8.505,15.8,85.3066731858115));
#44334=CARTESIAN_POINT('',(8.35603499314338,15.8,85.4390826561945));
#44335=CARTESIAN_POINT('Ctrl Pts',(8.505,15.8,85.3066731858115));
#44336=CARTESIAN_POINT('Ctrl Pts',(8.505,15.9179385772418,85.3066731858115));
#44337=CARTESIAN_POINT('Ctrl Pts',(8.54086304012327,16.0764310527784,85.3106030941529));
#44338=CARTESIAN_POINT('Ctrl Pts',(8.62145541370151,16.2176035248435,85.3181429539479));
#44339=CARTESIAN_POINT('Ctrl Pts',(8.64684940843773,16.2557977753682,85.3204017727898));
#44340=CARTESIAN_POINT('Ctrl Pts',(8.66003814345861,16.2744292787949,85.3215545492563));
#44341=CARTESIAN_POINT('Ctrl Pts',(8.67363423020825,16.2925558955514,85.3227195793178));
#44342=CARTESIAN_POINT('Ctrl Pts',(8.7205521873145,16.3514554569438,85.3266546996792));
#44343=CARTESIAN_POINT('Ctrl Pts',(8.77131943832023,16.4009043656078,85.3305312344449));
#44344=CARTESIAN_POINT('Ctrl Pts',(8.83055398400987,16.4462117636603,85.3344222728693));
#44345=CARTESIAN_POINT('Ctrl Pts',(8.8547843286754,16.4636679502074,85.3359553956004));
#44346=CARTESIAN_POINT('Ctrl Pts',(8.8861949024931,16.4843728290683,85.3378304187148));
#44347=CARTESIAN_POINT('Ctrl Pts',(8.92538849712145,16.5071421794607,85.3399698751664));
#44348=CARTESIAN_POINT('Ctrl Pts',(8.97938077241115,16.5345929028214,85.3426334541328));
#44349=CARTESIAN_POINT('Ctrl Pts',(9.03569842002898,16.5573899836454,85.3449477449916));
#44350=CARTESIAN_POINT('Ctrl Pts',(9.09316774712228,16.5752894292553,85.3468142604014));
#44351=CARTESIAN_POINT('Ctrl Pts',(9.23947932041198,16.611606923451,85.3506825029363));
#44352=CARTESIAN_POINT('Ctrl Pts',(9.36745606496479,16.6116832623999,85.3506959958052));
#44353=CARTESIAN_POINT('Ctrl Pts',(9.4866692068963,16.5851030550793,85.3478584147889));
#44354=CARTESIAN_POINT('Ctrl Pts',(9.49152112487657,16.5839940570477,85.3477402289228));
#44355=CARTESIAN_POINT('Ctrl Pts',(9.50001424450649,16.581993044702,85.3475272961553));
#44356=CARTESIAN_POINT('Ctrl Pts',(9.50970271448452,16.5795667525196,85.3472700502645));
#44357=CARTESIAN_POINT('Ctrl Pts',(9.51936951826886,16.5770017323372,85.3469991446667));
#44358=CARTESIAN_POINT('Ctrl Pts',(9.52902050818195,16.5743441772328,85.3467192253746));
#44359=CARTESIAN_POINT('Ctrl Pts',(9.55549383906246,16.5666555619593,85.3459127351656));
#44360=CARTESIAN_POINT('Ctrl Pts',(9.59840178362959,16.5520015558579,85.344396916677));
#44361=CARTESIAN_POINT('Ctrl Pts',(9.6540832365928,16.5281701476604,85.3420053250454));
#44362=CARTESIAN_POINT('Ctrl Pts',(9.72574555585249,16.4908918066207,85.3384036866979));
#44363=CARTESIAN_POINT('Ctrl Pts',(9.79253082541093,16.4459745469907,85.3343345112839));
#44364=CARTESIAN_POINT('Ctrl Pts',(9.85250976762847,16.3950350786248,85.3301373185125));
#44365=CARTESIAN_POINT('Ctrl Pts',(9.93483064967827,16.3144850829283,85.3239264410931));
#44366=CARTESIAN_POINT('Ctrl Pts',(10.0071745440962,16.2128038591041,85.3174382329924));
#44367=CARTESIAN_POINT('Ctrl Pts',(10.057758031708,16.0991078642724,85.3125075042899));
#44368=CARTESIAN_POINT('Ctrl Pts',(10.078672063003,16.0403516827864,85.3104115563631));
#44369=CARTESIAN_POINT('Ctrl Pts',(10.0949642083669,15.9803976278085,85.3087417687321));
#44370=CARTESIAN_POINT('Ctrl Pts',(10.1178006701332,15.8587378800666,85.3063526509483));
#44371=CARTESIAN_POINT('Ctrl Pts',(10.1182474458107,15.7215475976374,85.3063228611977));
#44372=CARTESIAN_POINT('Ctrl Pts',(10.0811386737492,15.5586344211364,85.310188833704));
#44373=CARTESIAN_POINT('Ctrl Pts',(10.0271730942457,15.4237431747111,85.3155709919468));
#44374=CARTESIAN_POINT('Ctrl Pts',(9.93612528575951,15.2840396015067,85.3238553111532));
#44375=CARTESIAN_POINT('Ctrl Pts',(9.83315711031573,15.1838884611021,85.3317387603146));
#44376=CARTESIAN_POINT('Ctrl Pts',(9.7346619221053,15.1144694922618,85.3378986529629));
#44377=CARTESIAN_POINT('Ctrl Pts',(9.6548195679892,15.0711281320789,85.342061878469));
#44378=CARTESIAN_POINT('Ctrl Pts',(9.5845744475483,15.0425478764307,85.3449563138224));
#44379=CARTESIAN_POINT('Ctrl Pts',(9.53780698901607,15.0280320991933,85.3464722484895));
#44380=CARTESIAN_POINT('Ctrl Pts',(9.51608572112935,15.0221025982153,85.3470971157239));
#44381=CARTESIAN_POINT('Ctrl Pts',(9.50519351381511,15.0192951792553,85.3473942354814));
#44382=CARTESIAN_POINT('Ctrl Pts',(9.49429929470381,15.0166439719612,85.3476758064351));
#44383=CARTESIAN_POINT('Ctrl Pts',(9.42858039309825,15.0016720477432,85.3492720117487));
#44384=CARTESIAN_POINT('Ctrl Pts',(9.31001561287879,14.9891031912116,85.3506669927535));
#44385=CARTESIAN_POINT('Ctrl Pts',(9.1803374115941,15.0028593633758,85.3491377784547));
#44386=CARTESIAN_POINT('Ctrl Pts',(9.09267762243124,15.0247228257435,85.3468147753307));
#44387=CARTESIAN_POINT('Ctrl Pts',(9.03520284211642,15.0426119288362,85.3449481349403));
#44388=CARTESIAN_POINT('Ctrl Pts',(8.96491506086939,15.0710987039933,85.3420566223853));
#44389=CARTESIAN_POINT('Ctrl Pts',(8.89830060869765,15.1074100272057,85.3385764674512));
#44390=CARTESIAN_POINT('Ctrl Pts',(8.84814018438728,15.1404381664927,85.3355833519254));
#44391=CARTESIAN_POINT('Ctrl Pts',(8.77601082966343,15.1941199284598,85.3309213351092));
#44392=CARTESIAN_POINT('Ctrl Pts',(8.7228233621219,15.246101550853,85.3268470112305));
#44393=CARTESIAN_POINT('Ctrl Pts',(8.68039050681583,15.2986562109445,85.3233064758915));
#44394=CARTESIAN_POINT('Ctrl Pts',(8.67111584921878,15.3104928289646,85.3225240350353));
#44395=CARTESIAN_POINT('Ctrl Pts',(8.65522068046374,15.3316550373053,85.3211613980828));
#44396=CARTESIAN_POINT('Ctrl Pts',(8.62502517013426,15.3757147794904,85.3184992676831));
#44397=CARTESIAN_POINT('Ctrl Pts',(8.54063322480884,15.5236112117938,85.310603260148));
#44398=CARTESIAN_POINT('Ctrl Pts',(8.505,15.6820614227582,85.3066731858115));
#44399=CARTESIAN_POINT('Ctrl Pts',(8.505,15.8,85.3066731858115));
#44400=CARTESIAN_POINT('Ctrl Pts',(8.35603499314338,15.8,85.4390826561945));
#44401=CARTESIAN_POINT('Ctrl Pts',(8.35603499314338,15.6627202519725,85.4390826561945));
#44402=CARTESIAN_POINT('Ctrl Pts',(8.39640281859525,15.4781780558787,85.4444905178981));
#44403=CARTESIAN_POINT('Ctrl Pts',(8.49372813179311,15.3037099876317,85.4554712250094));
#44404=CARTESIAN_POINT('Ctrl Pts',(8.52873347530619,15.2515214314165,85.4591853935954));
#44405=CARTESIAN_POINT('Ctrl Pts',(8.54720257389172,15.2263954689324,85.4610892717717));
#44406=CARTESIAN_POINT('Ctrl Pts',(8.55799266459696,15.2123260535644,85.4621833875471));
#44407=CARTESIAN_POINT('Ctrl Pts',(8.60739958396077,15.1498071578507,85.4671368089765));
#44408=CARTESIAN_POINT('Ctrl Pts',(8.66971693517491,15.0875063099098,85.4728628549599));
#44409=CARTESIAN_POINT('Ctrl Pts',(8.75499655724527,15.0226900205634,85.4794515057453));
#44410=CARTESIAN_POINT('Ctrl Pts',(8.81450469736164,14.9826783322091,85.4836911519947));
#44411=CARTESIAN_POINT('Ctrl Pts',(8.89391110377091,14.9384727132614,85.4886374013684));
#44412=CARTESIAN_POINT('Ctrl Pts',(8.97819116088274,14.903593487749,85.4927637202553));
#44413=CARTESIAN_POINT('Ctrl Pts',(9.04735019561901,14.8816229494821,85.4954334077506));
#44414=CARTESIAN_POINT('Ctrl Pts',(9.15304234143535,14.8547157047969,85.4987606437473));
#44415=CARTESIAN_POINT('Ctrl Pts',(9.31002212387416,14.8376927917007,85.5009593430419));
#44416=CARTESIAN_POINT('Ctrl Pts',(9.45354917166566,14.8532449033689,85.4989535397092));
#44417=CARTESIAN_POINT('Ctrl Pts',(9.53283457660932,14.8716784688763,85.4966665696332));
#44418=CARTESIAN_POINT('Ctrl Pts',(9.54597200279266,14.8749411777993,85.4962632794556));
#44419=CARTESIAN_POINT('Ctrl Pts',(9.55910119355026,14.8783947067353,85.4958378446216));
#44420=CARTESIAN_POINT('Ctrl Pts',(9.58527096084076,14.8856853198025,85.4949434208681));
#44421=CARTESIAN_POINT('Ctrl Pts',(9.64154714023013,14.9035142378301,85.4927752312384));
#44422=CARTESIAN_POINT('Ctrl Pts',(9.7257726708022,14.938502416334,85.48864489927));
#44423=CARTESIAN_POINT('Ctrl Pts',(9.82095295951565,14.9912740599348,85.4827275167418));
#44424=CARTESIAN_POINT('Ctrl Pts',(9.93758658799873,15.0752327539855,85.4740118542376));
#44425=CARTESIAN_POINT('Ctrl Pts',(10.0582364282556,15.1952877308291,85.4629318702328));
#44426=CARTESIAN_POINT('Ctrl Pts',(10.1635097686491,15.3605723341138,85.4513910623746));
#44427=CARTESIAN_POINT('Ctrl Pts',(10.2253511275564,15.5187131618124,85.4439361201402));
#44428=CARTESIAN_POINT('Ctrl Pts',(10.2676702177296,15.7087996732268,85.4385975861224));
#44429=CARTESIAN_POINT('Ctrl Pts',(10.2671411860703,15.8682847284844,85.4386400439914));
#44430=CARTESIAN_POINT('Ctrl Pts',(10.2411110001271,16.0101477612633,85.441938174718));
#44431=CARTESIAN_POINT('Ctrl Pts',(10.222497181123,16.0801829715165,85.4442465721495));
#44432=CARTESIAN_POINT('Ctrl Pts',(10.1985441116753,16.1489861273042,85.4471485778523));
#44433=CARTESIAN_POINT('Ctrl Pts',(10.140445547261,16.2824959491676,85.4539873067033));
#44434=CARTESIAN_POINT('Ctrl Pts',(10.0566824559075,16.4030718438372,85.4630358281122));
#44435=CARTESIAN_POINT('Ctrl Pts',(9.96015984107354,16.4995598748089,85.4717656307727));
#44436=CARTESIAN_POINT('Ctrl Pts',(9.88952955214136,16.5608297157303,85.477681416797));
#44437=CARTESIAN_POINT('Ctrl Pts',(9.81035193883595,16.6152393568737,85.4834442118835));
#44438=CARTESIAN_POINT('Ctrl Pts',(9.72483636139708,16.6606586538393,85.4885662989555));
#44439=CARTESIAN_POINT('Ctrl Pts',(9.65813475370038,16.6898037484486,85.4919764613753));
#44440=CARTESIAN_POINT('Ctrl Pts',(9.6065596797669,16.7077838948382,85.4941429373237));
#44441=CARTESIAN_POINT('Ctrl Pts',(9.5746828868594,16.7172323247418,85.4952968805524));
#44442=CARTESIAN_POINT('Ctrl Pts',(9.56305629792811,16.7204997032745,85.4956975301883));
#44443=CARTESIAN_POINT('Ctrl Pts',(9.55140693128475,16.7236542968834,85.4960853644285));
#44444=CARTESIAN_POINT('Ctrl Pts',(9.53972603545934,16.7266396251387,85.4964537623072));
#44445=CARTESIAN_POINT('Ctrl Pts',(9.52948187007311,16.7291027348195,85.4967587924218));
#44446=CARTESIAN_POINT('Ctrl Pts',(9.52362841368894,16.7304680703605,85.4969281164271));
#44447=CARTESIAN_POINT('Ctrl Pts',(9.37978678214075,16.7631990287376,85.5009941213014));
#44448=CARTESIAN_POINT('Ctrl Pts',(9.22435588573701,16.7630993137503,85.5009743602204));
#44449=CARTESIAN_POINT('Ctrl Pts',(9.04794555696647,16.7183902183462,85.4954326308204));
#44450=CARTESIAN_POINT('Ctrl Pts',(8.97879268762966,16.6964087072018,85.4927632839475));
#44451=CARTESIAN_POINT('Ctrl Pts',(8.91126359072523,16.6684953457075,85.489460606674));
#44452=CARTESIAN_POINT('Ctrl Pts',(8.84680287582055,16.6350364303463,85.4856715584966));
#44453=CARTESIAN_POINT('Ctrl Pts',(8.80015375962284,16.6073660501337,85.4826344158676));
#44454=CARTESIAN_POINT('Ctrl Pts',(8.76289021098275,16.5822842616593,85.4799785377766));
#44455=CARTESIAN_POINT('Ctrl Pts',(8.73421571262732,16.5611896429675,85.477810600089));
#44456=CARTESIAN_POINT('Ctrl Pts',(8.66423709283022,16.5065301286674,85.472314639594));
#44457=CARTESIAN_POINT('Ctrl Pts',(8.60474859865648,16.4472645215626,85.4668665636608));
#44458=CARTESIAN_POINT('Ctrl Pts',(8.55014120211907,16.3772240255913,85.4613625335412));
#44459=CARTESIAN_POINT('Ctrl Pts',(8.53434287032992,16.3557032208687,85.4597347029858));
#44460=CARTESIAN_POINT('Ctrl Pts',(8.51904255235788,16.333616011952,85.4581256707728));
#44461=CARTESIAN_POINT('Ctrl Pts',(8.48962600103117,16.2884083933886,85.4549757803719));
#44462=CARTESIAN_POINT('Ctrl Pts',(8.39668257439119,16.1218710106354,85.4444904181629));
#44463=CARTESIAN_POINT('Ctrl Pts',(8.35603499314338,15.9372797480275,85.4390826561945));
#44464=CARTESIAN_POINT('Ctrl Pts',(8.35603499314338,15.8,85.4390826561945));
#44465=CARTESIAN_POINT('Origin',(9.31,15.8,83.24125));
#44466=CARTESIAN_POINT('',(9.30971443151743,14.9950000506518,81.1524999870659));
#44467=CARTESIAN_POINT('',(8.50493382511065,15.8000495525908,81.0427739960352));
#44468=CARTESIAN_POINT('Ctrl Pts',(9.30971443151743,14.9950000506518,81.1524999870659));
#44469=CARTESIAN_POINT('Ctrl Pts',(9.47284767131029,14.9949421801988,81.1525147644529));
#44470=CARTESIAN_POINT('Ctrl Pts',(9.79584033527272,15.0993874455422,81.1239737564541));
#44471=CARTESIAN_POINT('Ctrl Pts',(10.0425595102383,15.4113740238506,81.0633302501805));
#44472=CARTESIAN_POINT('Ctrl Pts',(10.1189117455193,15.6998872287926,81.0414272750389));
#44473=CARTESIAN_POINT('Ctrl Pts',(10.1152364214667,15.99695011648,81.0423153895362));
#44474=CARTESIAN_POINT('Ctrl Pts',(10.0204956825243,16.2088719014764,81.0701904801504));
#44475=CARTESIAN_POINT('Ctrl Pts',(9.9044103854419,16.3436108471324,81.0944871436364));
#44476=CARTESIAN_POINT('Ctrl Pts',(9.88786634588363,16.361141904578,81.0977809418426));
#44477=CARTESIAN_POINT('Ctrl Pts',(9.80100095605804,16.4455527332759,81.1142474637718));
#44478=CARTESIAN_POINT('Ctrl Pts',(9.62439492967267,16.5644831932575,81.1417563388649));
#44479=CARTESIAN_POINT('Ctrl Pts',(9.38524990047136,16.6101492764359,81.1538705707198));
#44480=CARTESIAN_POINT('Ctrl Pts',(9.23365810330067,16.6027009170661,81.1519184980892));
#44481=CARTESIAN_POINT('Ctrl Pts',(9.12951062622373,16.5878157822367,81.1481620130899));
#44482=CARTESIAN_POINT('Ctrl Pts',(8.9511729466788,16.5345389475329,81.1348278227182));
#44483=CARTESIAN_POINT('Ctrl Pts',(8.8191656566872,16.4455872622242,81.1143735731117));
#44484=CARTESIAN_POINT('Ctrl Pts',(8.63368064477052,16.265506383372,81.0793273667541));
#44485=CARTESIAN_POINT('Ctrl Pts',(8.52785160642035,16.0691577161987,81.0488154213655));
#44486=CARTESIAN_POINT('Ctrl Pts',(8.50496051869156,15.8580350113622,81.0427179128319));
#44487=CARTESIAN_POINT('Ctrl Pts',(8.50493382511065,15.8000495525908,81.0427739960352));
#44488=CARTESIAN_POINT('Ctrl Pts',(8.50493382511065,15.8000495525908,81.0427739960352));
#44489=CARTESIAN_POINT('Ctrl Pts',(8.50489001938542,15.7048920282917,81.042866031847));
#44490=CARTESIAN_POINT('Ctrl Pts',(8.5487676875157,15.456580448563,81.0552684209999));
#44491=CARTESIAN_POINT('Ctrl Pts',(8.75653315952666,15.1754693805007,81.1086537222845));
#44492=CARTESIAN_POINT('Ctrl Pts',(9.05576289094108,15.0222450031167,81.1453157035286));
#44493=CARTESIAN_POINT('Ctrl Pts',(9.22496960714143,14.9950301133256,81.1524923104755));
#44494=CARTESIAN_POINT('Ctrl Pts',(9.30971443151743,14.9950000506518,81.1524999870659));
#44495=CARTESIAN_POINT('',(8.505,15.8,83.24125));
#44496=CARTESIAN_POINT('Origin',(9.31,18.775,78.));
#44497=CARTESIAN_POINT('',(1.81,14.25,78.));
#44498=CARTESIAN_POINT('Origin',(9.31,14.25,78.));
#44499=CARTESIAN_POINT('',(1.81,17.5,78.));
#44500=CARTESIAN_POINT('',(1.81,18.775,78.));
#44501=CARTESIAN_POINT('',(1.81,20.5,78.));
#44502=CARTESIAN_POINT('Ctrl Pts',(1.81,17.5,78.));
#44503=CARTESIAN_POINT('Ctrl Pts',(1.81,17.5,77.905556478434));
#44504=CARTESIAN_POINT('Ctrl Pts',(1.81183067420966,17.5090634188645,77.8079678203077));
#44505=CARTESIAN_POINT('Ctrl Pts',(1.81931072941389,17.5471495606178,77.6140027878517));
#44506=CARTESIAN_POINT('Ctrl Pts',(1.82495532590085,17.5761632619054,77.5176244577088));
#44507=CARTESIAN_POINT('Ctrl Pts',(1.84624979272205,17.6910934876829,77.2405577082036));
#44508=CARTESIAN_POINT('Ctrl Pts',(1.86639493542522,17.806452793408,77.0722268630324));
#44509=CARTESIAN_POINT('Ctrl Pts',(1.90436372347101,18.0722343097285,76.8064453467119));
#44510=CARTESIAN_POINT('Ctrl Pts',(1.92468773810844,18.2405619924549,76.6910918735274));
#44511=CARTESIAN_POINT('Ctrl Pts',(1.94629082256958,18.5176204988066,76.5761648226022));
#44512=CARTESIAN_POINT('Ctrl Pts',(1.95203778940752,18.6139962349031,76.547151319492));
#44513=CARTESIAN_POINT('Ctrl Pts',(1.9596606794129,18.8079605728532,76.5090643698119));
#44514=CARTESIAN_POINT('Ctrl Pts',(1.96153077165046,18.9055511860275,76.5));
#44515=CARTESIAN_POINT('Ctrl Pts',(1.96153077165046,19.0944488139725,76.5));
#44516=CARTESIAN_POINT('Ctrl Pts',(1.9596606794129,19.1920394271468,76.5090643698119));
#44517=CARTESIAN_POINT('Ctrl Pts',(1.95203778940752,19.3860037650969,76.547151319492));
#44518=CARTESIAN_POINT('Ctrl Pts',(1.94629082256958,19.4823795011934,76.5761648226022));
#44519=CARTESIAN_POINT('Ctrl Pts',(1.92468773810844,19.7594380075451,76.6910918735274));
#44520=CARTESIAN_POINT('Ctrl Pts',(1.90436372347101,19.9277656902715,76.8064453467119));
#44521=CARTESIAN_POINT('Ctrl Pts',(1.86639493542522,20.193547206592,77.0722268630324));
#44522=CARTESIAN_POINT('Ctrl Pts',(1.84624979272205,20.3089065123171,77.2405577082036));
#44523=CARTESIAN_POINT('Ctrl Pts',(1.82495532590085,20.4238367380946,77.5176244577088));
#44524=CARTESIAN_POINT('Ctrl Pts',(1.81931072941389,20.4528504393822,77.6140027878517));
#44525=CARTESIAN_POINT('Ctrl Pts',(1.81183067420965,20.4909365811355,77.8079678203077));
#44526=CARTESIAN_POINT('Ctrl Pts',(1.81,20.5,77.905556478434));
#44527=CARTESIAN_POINT('Ctrl Pts',(1.81,20.5,78.));
#44528=CARTESIAN_POINT('',(1.81,23.3,78.));
#44529=CARTESIAN_POINT('',(1.81,18.775,78.));
#44530=CARTESIAN_POINT('Origin',(9.31,23.3,78.));
#44531=CARTESIAN_POINT('',(1.96153077165046,19.,79.5));
#44532=CARTESIAN_POINT('Ctrl Pts',(1.81,20.5,78.));
#44533=CARTESIAN_POINT('Ctrl Pts',(1.81,20.5,78.094443521566));
#44534=CARTESIAN_POINT('Ctrl Pts',(1.81183067420966,20.4909365811355,78.1920321796923));
#44535=CARTESIAN_POINT('Ctrl Pts',(1.81931072941389,20.4528504393822,78.3859972121483));
#44536=CARTESIAN_POINT('Ctrl Pts',(1.82495532590085,20.4238367380946,78.4823755422912));
#44537=CARTESIAN_POINT('Ctrl Pts',(1.84624979272205,20.3089065123171,78.7594422917964));
#44538=CARTESIAN_POINT('Ctrl Pts',(1.86639493542522,20.193547206592,78.9277731369676));
#44539=CARTESIAN_POINT('Ctrl Pts',(1.90436372347101,19.9277656902715,79.1935546532881));
#44540=CARTESIAN_POINT('Ctrl Pts',(1.92468773810844,19.7594380075451,79.3089081264726));
#44541=CARTESIAN_POINT('Ctrl Pts',(1.94629082256958,19.4823795011934,79.4238351773978));
#44542=CARTESIAN_POINT('Ctrl Pts',(1.95203778940752,19.3860037650969,79.452848680508));
#44543=CARTESIAN_POINT('Ctrl Pts',(1.9596606794129,19.1920394271468,79.4909356301881));
#44544=CARTESIAN_POINT('Ctrl Pts',(1.96153077165046,19.0944488139725,79.5));
#44545=CARTESIAN_POINT('Ctrl Pts',(1.96153077165046,19.,79.5));
#44546=CARTESIAN_POINT('Ctrl Pts',(1.96153077165046,19.,79.5));
#44547=CARTESIAN_POINT('Ctrl Pts',(1.96153077165046,18.9055511860275,79.5));
#44548=CARTESIAN_POINT('Ctrl Pts',(1.9596606794129,18.8079605728532,79.4909356301881));
#44549=CARTESIAN_POINT('Ctrl Pts',(1.95203778940752,18.6139962349031,79.452848680508));
#44550=CARTESIAN_POINT('Ctrl Pts',(1.94629082256958,18.5176204988066,79.4238351773978));
#44551=CARTESIAN_POINT('Ctrl Pts',(1.92468773810844,18.2405619924549,79.3089081264726));
#44552=CARTESIAN_POINT('Ctrl Pts',(1.90436372347101,18.0722343097285,79.1935546532881));
#44553=CARTESIAN_POINT('Ctrl Pts',(1.86639493542522,17.806452793408,78.9277731369676));
#44554=CARTESIAN_POINT('Ctrl Pts',(1.84624979272205,17.6910934876829,78.7594422917964));
#44555=CARTESIAN_POINT('Ctrl Pts',(1.82495532590085,17.5761632619054,78.4823755422912));
#44556=CARTESIAN_POINT('Ctrl Pts',(1.81931072941389,17.5471495606178,78.3859972121483));
#44557=CARTESIAN_POINT('Ctrl Pts',(1.81183067420966,17.5090634188645,78.1920321796923));
#44558=CARTESIAN_POINT('Ctrl Pts',(1.81,17.5,78.0944435215661));
#44559=CARTESIAN_POINT('Ctrl Pts',(1.81,17.5,78.));
#44560=CARTESIAN_POINT('',(16.6584692283495,19.,76.5));
#44561=CARTESIAN_POINT('Ctrl Pts',(16.6584692283495,19.,76.5));
#44562=CARTESIAN_POINT('Ctrl Pts',(16.6584692283495,18.9055511860275,76.5));
#44563=CARTESIAN_POINT('Ctrl Pts',(16.6603393205871,18.8079605728532,76.5090643698119));
#44564=CARTESIAN_POINT('Ctrl Pts',(16.6679622105925,18.6139962349031,76.547151319492));
#44565=CARTESIAN_POINT('Ctrl Pts',(16.6737091774304,18.5176204988066,76.5761648226022));
#44566=CARTESIAN_POINT('Ctrl Pts',(16.6953122618916,18.2405619924549,76.6910918735274));
#44567=CARTESIAN_POINT('Ctrl Pts',(16.715636276529,18.0722343097285,76.8064453467119));
#44568=CARTESIAN_POINT('Ctrl Pts',(16.7536050645748,17.806452793408,77.0722268630324));
#44569=CARTESIAN_POINT('Ctrl Pts',(16.773750207278,17.6910934876829,77.2405577082036));
#44570=CARTESIAN_POINT('Ctrl Pts',(16.7950446740992,17.5761632619054,77.5176244577088));
#44571=CARTESIAN_POINT('Ctrl Pts',(16.8006892705861,17.5471495606178,77.6140027878517));
#44572=CARTESIAN_POINT('Ctrl Pts',(16.8081693257903,17.5090634188645,77.8079678203077));
#44573=CARTESIAN_POINT('Ctrl Pts',(16.81,17.5,77.905556478434));
#44574=CARTESIAN_POINT('Ctrl Pts',(16.81,17.5,78.094443521566));
#44575=CARTESIAN_POINT('Ctrl Pts',(16.8081693257903,17.5090634188645,78.1920321796923));
#44576=CARTESIAN_POINT('Ctrl Pts',(16.8006892705861,17.5471495606178,78.3859972121484));
#44577=CARTESIAN_POINT('Ctrl Pts',(16.7950446740992,17.5761632619054,78.4823755422912));
#44578=CARTESIAN_POINT('Ctrl Pts',(16.773750207278,17.6910934876829,78.7594422917964));
#44579=CARTESIAN_POINT('Ctrl Pts',(16.7536050645748,17.806452793408,78.9277731369676));
#44580=CARTESIAN_POINT('Ctrl Pts',(16.715636276529,18.0722343097285,79.1935546532881));
#44581=CARTESIAN_POINT('Ctrl Pts',(16.6953122618916,18.2405619924549,79.3089081264726));
#44582=CARTESIAN_POINT('Ctrl Pts',(16.6737091774304,18.5176204988066,79.4238351773978));
#44583=CARTESIAN_POINT('Ctrl Pts',(16.6679622105925,18.6139962349031,79.452848680508));
#44584=CARTESIAN_POINT('Ctrl Pts',(16.6603393205871,18.8079605728532,79.4909356301881));
#44585=CARTESIAN_POINT('Ctrl Pts',(16.6584692283495,18.9055511860275,79.5));
#44586=CARTESIAN_POINT('Ctrl Pts',(16.6584692283495,19.0944488139725,79.5));
#44587=CARTESIAN_POINT('Ctrl Pts',(16.6603393205871,19.1920394271468,79.4909356301881));
#44588=CARTESIAN_POINT('Ctrl Pts',(16.6679622105925,19.3860037650969,79.452848680508));
#44589=CARTESIAN_POINT('Ctrl Pts',(16.6737091774304,19.4823795011934,79.4238351773978));
#44590=CARTESIAN_POINT('Ctrl Pts',(16.6953122618916,19.7594380075451,79.3089081264726));
#44591=CARTESIAN_POINT('Ctrl Pts',(16.715636276529,19.9277656902715,79.1935546532881));
#44592=CARTESIAN_POINT('Ctrl Pts',(16.7536050645748,20.193547206592,78.9277731369676));
#44593=CARTESIAN_POINT('Ctrl Pts',(16.7737502072779,20.3089065123171,78.7594422917965));
#44594=CARTESIAN_POINT('Ctrl Pts',(16.7950446740991,20.4238367380946,78.4823755422912));
#44595=CARTESIAN_POINT('Ctrl Pts',(16.8006892705861,20.4528504393822,78.3859972121483));
#44596=CARTESIAN_POINT('Ctrl Pts',(16.8081693257903,20.4909365811355,78.1920321796923));
#44597=CARTESIAN_POINT('Ctrl Pts',(16.81,20.5,78.094443521566));
#44598=CARTESIAN_POINT('Ctrl Pts',(16.81,20.5,77.905556478434));
#44599=CARTESIAN_POINT('Ctrl Pts',(16.8081693257903,20.4909365811355,77.8079678203077));
#44600=CARTESIAN_POINT('Ctrl Pts',(16.8006892705861,20.4528504393822,77.6140027878517));
#44601=CARTESIAN_POINT('Ctrl Pts',(16.7950446740992,20.4238367380946,77.5176244577088));
#44602=CARTESIAN_POINT('Ctrl Pts',(16.773750207278,20.3089065123172,77.2405577082036));
#44603=CARTESIAN_POINT('Ctrl Pts',(16.7536050645748,20.193547206592,77.0722268630324));
#44604=CARTESIAN_POINT('Ctrl Pts',(16.715636276529,19.9277656902715,76.8064453467119));
#44605=CARTESIAN_POINT('Ctrl Pts',(16.6953122618916,19.7594380075451,76.6910918735274));
#44606=CARTESIAN_POINT('Ctrl Pts',(16.6737091774304,19.4823795011934,76.5761648226022));
#44607=CARTESIAN_POINT('Ctrl Pts',(16.6679622105925,19.3860037650969,76.547151319492));
#44608=CARTESIAN_POINT('Ctrl Pts',(16.6603393205871,19.1920394271468,76.5090643698119));
#44609=CARTESIAN_POINT('Ctrl Pts',(16.6584692283495,19.0944488139725,76.5));
#44610=CARTESIAN_POINT('Ctrl Pts',(16.6584692283495,19.,76.5));
#44611=CARTESIAN_POINT('',(14.2832727198514,19.,83.6139610306789));
#44612=CARTESIAN_POINT('Ctrl Pts',(14.2832727198514,19.,83.6139610306789));
#44613=CARTESIAN_POINT('Ctrl Pts',(14.2832727198514,18.9055511860275,83.6139610306789));
#44614=CARTESIAN_POINT('Ctrl Pts',(14.2763577914438,18.8079605728532,83.62011276297));
#44615=CARTESIAN_POINT('Ctrl Pts',(14.2471849704709,18.6139962349031,83.645757854205));
#44616=CARTESIAN_POINT('Ctrl Pts',(14.2249320231437,18.5176204988066,83.6652416250364));
#44617=CARTESIAN_POINT('Ctrl Pts',(14.1362038196909,18.2405619924549,83.7414139704425));
#44618=CARTESIAN_POINT('Ctrl Pts',(14.0464667888171,18.0722343097285,83.8166918200176));
#44619=CARTESIAN_POINT('Ctrl Pts',(13.8352776378501,17.806452793408,83.9824645131764));
#44620=CARTESIAN_POINT('Ctrl Pts',(13.699571421043,17.6910934876829,84.0840761411059));
#44621=CARTESIAN_POINT('Ctrl Pts',(13.4702718108381,17.5761632619054,84.2410510650857));
#44622=CARTESIAN_POINT('Ctrl Pts',(13.3896280268035,17.5471495606178,84.2941285941089));
#44623=CARTESIAN_POINT('Ctrl Pts',(13.2253894088528,17.5090634188645,84.3975890281656));
#44624=CARTESIAN_POINT('Ctrl Pts',(13.1417904888991,17.5,84.4479687676003));
#44625=CARTESIAN_POINT('Ctrl Pts',(12.9782095111009,17.5,84.5424122891663));
#44626=CARTESIAN_POINT('Ctrl Pts',(12.8927799169376,17.5090634188645,84.5896212078578));
#44627=CARTESIAN_POINT('Ctrl Pts',(12.7210612437826,17.5471495606178,84.6801258062573));
#44628=CARTESIAN_POINT('Ctrl Pts',(12.6347728632611,17.5761632619054,84.7234266073769));
#44629=CARTESIAN_POINT('Ctrl Pts',(12.384178786235,17.6910934876829,84.8435184329023));
#44630=CARTESIAN_POINT('Ctrl Pts',(12.2283274267246,17.806452793408,84.9102376501441));
#44631=CARTESIAN_POINT('Ctrl Pts',(11.9791694877118,18.0722343097285,85.0102464733058));
#44632=CARTESIAN_POINT('Ctrl Pts',(11.8691084422006,18.2405619924549,85.0503220969151));
#44633=CARTESIAN_POINT('Ctrl Pts',(11.7587771542868,18.5176204988066,85.0890768024343));
#44634=CARTESIAN_POINT('Ctrl Pts',(11.7307772401216,18.6139962349031,85.098606534713));
#44635=CARTESIAN_POINT('Ctrl Pts',(11.6939815291433,18.8079605728532,85.1110483931581));
#44636=CARTESIAN_POINT('Ctrl Pts',(11.6851965084981,18.9055511860275,85.1139610306789));
#44637=CARTESIAN_POINT('Ctrl Pts',(11.6851965084981,19.0944488139725,85.1139610306789));
#44638=CARTESIAN_POINT('Ctrl Pts',(11.6939815291433,19.1920394271468,85.1110483931581));
#44639=CARTESIAN_POINT('Ctrl Pts',(11.7307772401216,19.3860037650969,85.098606534713));
#44640=CARTESIAN_POINT('Ctrl Pts',(11.7587771542868,19.4823795011934,85.0890768024343));
#44641=CARTESIAN_POINT('Ctrl Pts',(11.8691084422006,19.7594380075451,85.0503220969151));
#44642=CARTESIAN_POINT('Ctrl Pts',(11.9791694877118,19.9277656902715,85.0102464733058));
#44643=CARTESIAN_POINT('Ctrl Pts',(12.2283274267246,20.193547206592,84.9102376501441));
#44644=CARTESIAN_POINT('Ctrl Pts',(12.384178786235,20.3089065123171,84.8435184329023));
#44645=CARTESIAN_POINT('Ctrl Pts',(12.6347728632611,20.4238367380946,84.7234266073769));
#44646=CARTESIAN_POINT('Ctrl Pts',(12.7210612437826,20.4528504393822,84.6801258062573));
#44647=CARTESIAN_POINT('Ctrl Pts',(12.8927799169376,20.4909365811355,84.5896212078578));
#44648=CARTESIAN_POINT('Ctrl Pts',(12.9782095111009,20.5,84.5424122891663));
#44649=CARTESIAN_POINT('Ctrl Pts',(13.1417904888991,20.5,84.4479687676003));
#44650=CARTESIAN_POINT('Ctrl Pts',(13.2253894088528,20.4909365811355,84.3975890281656));
#44651=CARTESIAN_POINT('Ctrl Pts',(13.3896280268035,20.4528504393822,84.2941285941089));
#44652=CARTESIAN_POINT('Ctrl Pts',(13.4702718108381,20.4238367380946,84.2410510650857));
#44653=CARTESIAN_POINT('Ctrl Pts',(13.699571421043,20.3089065123171,84.0840761411059));
#44654=CARTESIAN_POINT('Ctrl Pts',(13.8352776378501,20.193547206592,83.9824645131764));
#44655=CARTESIAN_POINT('Ctrl Pts',(14.0464667888171,19.9277656902715,83.8166918200176));
#44656=CARTESIAN_POINT('Ctrl Pts',(14.1362038196909,19.7594380075451,83.7414139704425));
#44657=CARTESIAN_POINT('Ctrl Pts',(14.2249320231437,19.4823795011934,83.6652416250364));
#44658=CARTESIAN_POINT('Ctrl Pts',(14.2471849704709,19.3860037650969,83.645757854205));
#44659=CARTESIAN_POINT('Ctrl Pts',(14.2763577914438,19.1920394271468,83.62011276297));
#44660=CARTESIAN_POINT('Ctrl Pts',(14.2832727198514,19.0944488139725,83.6139610306789));
#44661=CARTESIAN_POINT('Ctrl Pts',(14.2832727198514,19.,83.6139610306789));
#44662=CARTESIAN_POINT('',(6.93480349150189,19.,85.1139610306789));
#44663=CARTESIAN_POINT('Ctrl Pts',(6.93480349150189,19.,85.1139610306789));
#44664=CARTESIAN_POINT('Ctrl Pts',(6.93480349150189,18.9055511860275,85.1139610306789));
#44665=CARTESIAN_POINT('Ctrl Pts',(6.92601847085671,18.8079605728532,85.1110483931581));
#44666=CARTESIAN_POINT('Ctrl Pts',(6.88922275987842,18.6139962349031,85.098606534713));
#44667=CARTESIAN_POINT('Ctrl Pts',(6.86122284571324,18.5176204988066,85.0890768024343));
#44668=CARTESIAN_POINT('Ctrl Pts',(6.75089155779936,18.2405619924549,85.0503220969151));
#44669=CARTESIAN_POINT('Ctrl Pts',(6.64083051228816,18.0722343097285,85.0102464733058));
#44670=CARTESIAN_POINT('Ctrl Pts',(6.39167257327537,17.806452793408,84.9102376501441));
#44671=CARTESIAN_POINT('Ctrl Pts',(6.23582121376502,17.6910934876829,84.8435184329023));
#44672=CARTESIAN_POINT('Ctrl Pts',(5.98522713673891,17.5761632619054,84.7234266073769));
#44673=CARTESIAN_POINT('Ctrl Pts',(5.89893875621735,17.5471495606178,84.6801258062573));
#44674=CARTESIAN_POINT('Ctrl Pts',(5.72722008306242,17.5090634188645,84.5896212078578));
#44675=CARTESIAN_POINT('Ctrl Pts',(5.64179048889907,17.5,84.5424122891663));
#44676=CARTESIAN_POINT('Ctrl Pts',(5.47820951110094,17.5,84.4479687676003));
#44677=CARTESIAN_POINT('Ctrl Pts',(5.39461059114724,17.5090634188645,84.3975890281656));
#44678=CARTESIAN_POINT('Ctrl Pts',(5.23037197319652,17.5471495606178,84.2941285941089));
#44679=CARTESIAN_POINT('Ctrl Pts',(5.14972818916194,17.5761632619054,84.2410510650857));
#44680=CARTESIAN_POINT('Ctrl Pts',(4.92042857895703,17.6910934876829,84.0840761411059));
#44681=CARTESIAN_POINT('Ctrl Pts',(4.78472236214986,17.806452793408,83.9824645131764));
#44682=CARTESIAN_POINT('Ctrl Pts',(4.57353321118285,18.0722343097285,83.8166918200176));
#44683=CARTESIAN_POINT('Ctrl Pts',(4.48379618030908,18.2405619924549,83.7414139704425));
#44684=CARTESIAN_POINT('Ctrl Pts',(4.39506797685635,18.5176204988066,83.6652416250364));
#44685=CARTESIAN_POINT('Ctrl Pts',(4.3728150295291,18.6139962349031,83.645757854205));
#44686=CARTESIAN_POINT('Ctrl Pts',(4.34364220855619,18.8079605728532,83.62011276297));
#44687=CARTESIAN_POINT('Ctrl Pts',(4.33672728014858,18.9055511860275,83.6139610306789));
#44688=CARTESIAN_POINT('Ctrl Pts',(4.33672728014858,19.0944488139725,83.6139610306789));
#44689=CARTESIAN_POINT('Ctrl Pts',(4.34364220855619,19.1920394271468,83.62011276297));
#44690=CARTESIAN_POINT('Ctrl Pts',(4.3728150295291,19.3860037650969,83.645757854205));
#44691=CARTESIAN_POINT('Ctrl Pts',(4.39506797685635,19.4823795011934,83.6652416250364));
#44692=CARTESIAN_POINT('Ctrl Pts',(4.48379618030908,19.7594380075451,83.7414139704425));
#44693=CARTESIAN_POINT('Ctrl Pts',(4.57353321118285,19.9277656902715,83.8166918200176));
#44694=CARTESIAN_POINT('Ctrl Pts',(4.78472236214986,20.193547206592,83.9824645131764));
#44695=CARTESIAN_POINT('Ctrl Pts',(4.92042857895703,20.3089065123171,84.0840761411059));
#44696=CARTESIAN_POINT('Ctrl Pts',(5.14972818916194,20.4238367380946,84.2410510650857));
#44697=CARTESIAN_POINT('Ctrl Pts',(5.23037197319652,20.4528504393822,84.2941285941089));
#44698=CARTESIAN_POINT('Ctrl Pts',(5.39461059114724,20.4909365811355,84.3975890281656));
#44699=CARTESIAN_POINT('Ctrl Pts',(5.47820951110094,20.5,84.4479687676003));
#44700=CARTESIAN_POINT('Ctrl Pts',(5.64179048889906,20.5,84.5424122891663));
#44701=CARTESIAN_POINT('Ctrl Pts',(5.72722008306241,20.4909365811355,84.5896212078578));
#44702=CARTESIAN_POINT('Ctrl Pts',(5.89893875621735,20.4528504393822,84.6801258062573));
#44703=CARTESIAN_POINT('Ctrl Pts',(5.98522713673891,20.4238367380946,84.7234266073769));
#44704=CARTESIAN_POINT('Ctrl Pts',(6.23582121376502,20.3089065123171,84.8435184329023));
#44705=CARTESIAN_POINT('Ctrl Pts',(6.39167257327537,20.193547206592,84.9102376501441));
#44706=CARTESIAN_POINT('Ctrl Pts',(6.64083051228816,19.9277656902715,85.0102464733058));
#44707=CARTESIAN_POINT('Ctrl Pts',(6.75089155779936,19.7594380075451,85.0503220969151));
#44708=CARTESIAN_POINT('Ctrl Pts',(6.86122284571324,19.4823795011934,85.0890768024343));
#44709=CARTESIAN_POINT('Ctrl Pts',(6.88922275987842,19.3860037650969,85.098606534713));
#44710=CARTESIAN_POINT('Ctrl Pts',(6.92601847085671,19.1920394271468,85.1110483931581));
#44711=CARTESIAN_POINT('Ctrl Pts',(6.93480349150189,19.0944488139725,85.1139610306789));
#44712=CARTESIAN_POINT('Ctrl Pts',(6.93480349150189,19.,85.1139610306789));
#44713=CARTESIAN_POINT('',(4.33672728014858,19.,72.3860389693211));
#44714=CARTESIAN_POINT('Ctrl Pts',(4.33672728014858,19.,72.3860389693211));
#44715=CARTESIAN_POINT('Ctrl Pts',(4.33672728014858,18.9055511860275,72.3860389693211));
#44716=CARTESIAN_POINT('Ctrl Pts',(4.34364220855619,18.8079605728532,72.37988723703));
#44717=CARTESIAN_POINT('Ctrl Pts',(4.3728150295291,18.6139962349031,72.354242145795));
#44718=CARTESIAN_POINT('Ctrl Pts',(4.39506797685635,18.5176204988066,72.3347583749636));
#44719=CARTESIAN_POINT('Ctrl Pts',(4.48379618030908,18.2405619924549,72.2585860295575));
#44720=CARTESIAN_POINT('Ctrl Pts',(4.57353321118286,18.0722343097285,72.1833081799824));
#44721=CARTESIAN_POINT('Ctrl Pts',(4.78472236214986,17.806452793408,72.0175354868236));
#44722=CARTESIAN_POINT('Ctrl Pts',(4.92042857895703,17.6910934876829,71.9159238588941));
#44723=CARTESIAN_POINT('Ctrl Pts',(5.14972818916194,17.5761632619054,71.7589489349143));
#44724=CARTESIAN_POINT('Ctrl Pts',(5.23037197319652,17.5471495606178,71.7058714058911));
#44725=CARTESIAN_POINT('Ctrl Pts',(5.39461059114724,17.5090634188645,71.6024109718344));
#44726=CARTESIAN_POINT('Ctrl Pts',(5.47820951110094,17.5,71.5520312323997));
#44727=CARTESIAN_POINT('Ctrl Pts',(5.64179048889907,17.5,71.4575877108337));
#44728=CARTESIAN_POINT('Ctrl Pts',(5.72722008306241,17.5090634188645,71.4103787921422));
#44729=CARTESIAN_POINT('Ctrl Pts',(5.89893875621735,17.5471495606178,71.3198741937427));
#44730=CARTESIAN_POINT('Ctrl Pts',(5.98522713673891,17.5761632619054,71.2765733926231));
#44731=CARTESIAN_POINT('Ctrl Pts',(6.23582121376502,17.6910934876829,71.1564815670977));
#44732=CARTESIAN_POINT('Ctrl Pts',(6.39167257327537,17.806452793408,71.0897623498559));
#44733=CARTESIAN_POINT('Ctrl Pts',(6.64083051228816,18.0722343097285,70.9897535266942));
#44734=CARTESIAN_POINT('Ctrl Pts',(6.75089155779937,18.2405619924549,70.9496779030849));
#44735=CARTESIAN_POINT('Ctrl Pts',(6.86122284571324,18.5176204988066,70.9109231975657));
#44736=CARTESIAN_POINT('Ctrl Pts',(6.88922275987843,18.6139962349031,70.901393465287));
#44737=CARTESIAN_POINT('Ctrl Pts',(6.92601847085672,18.8079605728532,70.8889516068419));
#44738=CARTESIAN_POINT('Ctrl Pts',(6.93480349150189,18.9055511860275,70.8860389693211));
#44739=CARTESIAN_POINT('Ctrl Pts',(6.93480349150189,19.0944488139725,70.8860389693211));
#44740=CARTESIAN_POINT('Ctrl Pts',(6.92601847085672,19.1920394271468,70.8889516068419));
#44741=CARTESIAN_POINT('Ctrl Pts',(6.88922275987843,19.3860037650969,70.901393465287));
#44742=CARTESIAN_POINT('Ctrl Pts',(6.86122284571324,19.4823795011934,70.9109231975657));
#44743=CARTESIAN_POINT('Ctrl Pts',(6.75089155779936,19.7594380075451,70.9496779030849));
#44744=CARTESIAN_POINT('Ctrl Pts',(6.64083051228816,19.9277656902715,70.9897535266942));
#44745=CARTESIAN_POINT('Ctrl Pts',(6.39167257327537,20.193547206592,71.0897623498559));
#44746=CARTESIAN_POINT('Ctrl Pts',(6.23582121376502,20.3089065123171,71.1564815670977));
#44747=CARTESIAN_POINT('Ctrl Pts',(5.9852271367389,20.4238367380946,71.2765733926231));
#44748=CARTESIAN_POINT('Ctrl Pts',(5.89893875621735,20.4528504393822,71.3198741937427));
#44749=CARTESIAN_POINT('Ctrl Pts',(5.72722008306241,20.4909365811355,71.4103787921422));
#44750=CARTESIAN_POINT('Ctrl Pts',(5.64179048889907,20.5,71.4575877108337));
#44751=CARTESIAN_POINT('Ctrl Pts',(5.47820951110094,20.5,71.5520312323997));
#44752=CARTESIAN_POINT('Ctrl Pts',(5.39461059114724,20.4909365811355,71.6024109718344));
#44753=CARTESIAN_POINT('Ctrl Pts',(5.23037197319652,20.4528504393822,71.7058714058911));
#44754=CARTESIAN_POINT('Ctrl Pts',(5.14972818916194,20.4238367380946,71.7589489349143));
#44755=CARTESIAN_POINT('Ctrl Pts',(4.92042857895703,20.3089065123171,71.9159238588941));
#44756=CARTESIAN_POINT('Ctrl Pts',(4.78472236214986,20.193547206592,72.0175354868236));
#44757=CARTESIAN_POINT('Ctrl Pts',(4.57353321118286,19.9277656902715,72.1833081799824));
#44758=CARTESIAN_POINT('Ctrl Pts',(4.48379618030908,19.7594380075451,72.2585860295575));
#44759=CARTESIAN_POINT('Ctrl Pts',(4.39506797685635,19.4823795011934,72.3347583749636));
#44760=CARTESIAN_POINT('Ctrl Pts',(4.3728150295291,19.3860037650969,72.354242145795));
#44761=CARTESIAN_POINT('Ctrl Pts',(4.34364220855619,19.1920394271468,72.37988723703));
#44762=CARTESIAN_POINT('Ctrl Pts',(4.33672728014858,19.0944488139725,72.3860389693211));
#44763=CARTESIAN_POINT('Ctrl Pts',(4.33672728014858,19.,72.3860389693211));
#44764=CARTESIAN_POINT('',(11.6851965084981,19.,70.8860389693211));
#44765=CARTESIAN_POINT('Ctrl Pts',(11.6851965084981,19.,70.8860389693211));
#44766=CARTESIAN_POINT('Ctrl Pts',(11.6851965084981,18.9055511860275,70.8860389693211));
#44767=CARTESIAN_POINT('Ctrl Pts',(11.6939815291433,18.8079605728532,70.8889516068419));
#44768=CARTESIAN_POINT('Ctrl Pts',(11.7307772401216,18.6139962349031,70.901393465287));
#44769=CARTESIAN_POINT('Ctrl Pts',(11.7587771542868,18.5176204988066,70.9109231975657));
#44770=CARTESIAN_POINT('Ctrl Pts',(11.8691084422006,18.2405619924549,70.9496779030849));
#44771=CARTESIAN_POINT('Ctrl Pts',(11.9791694877118,18.0722343097285,70.9897535266942));
#44772=CARTESIAN_POINT('Ctrl Pts',(12.2283274267246,17.806452793408,71.0897623498559));
#44773=CARTESIAN_POINT('Ctrl Pts',(12.384178786235,17.6910934876829,71.1564815670977));
#44774=CARTESIAN_POINT('Ctrl Pts',(12.6347728632611,17.5761632619054,71.2765733926231));
#44775=CARTESIAN_POINT('Ctrl Pts',(12.7210612437826,17.5471495606178,71.3198741937427));
#44776=CARTESIAN_POINT('Ctrl Pts',(12.8927799169376,17.5090634188645,71.4103787921422));
#44777=CARTESIAN_POINT('Ctrl Pts',(12.9782095111009,17.5,71.4575877108337));
#44778=CARTESIAN_POINT('Ctrl Pts',(13.1417904888991,17.5,71.5520312323997));
#44779=CARTESIAN_POINT('Ctrl Pts',(13.2253894088528,17.5090634188645,71.6024109718344));
#44780=CARTESIAN_POINT('Ctrl Pts',(13.3896280268035,17.5471495606178,71.7058714058911));
#44781=CARTESIAN_POINT('Ctrl Pts',(13.4702718108381,17.5761632619054,71.7589489349143));
#44782=CARTESIAN_POINT('Ctrl Pts',(13.699571421043,17.6910934876829,71.9159238588941));
#44783=CARTESIAN_POINT('Ctrl Pts',(13.8352776378501,17.806452793408,72.0175354868236));
#44784=CARTESIAN_POINT('Ctrl Pts',(14.0464667888171,18.0722343097285,72.1833081799824));
#44785=CARTESIAN_POINT('Ctrl Pts',(14.1362038196909,18.2405619924549,72.2585860295575));
#44786=CARTESIAN_POINT('Ctrl Pts',(14.2249320231436,18.5176204988066,72.3347583749636));
#44787=CARTESIAN_POINT('Ctrl Pts',(14.2471849704709,18.6139962349031,72.354242145795));
#44788=CARTESIAN_POINT('Ctrl Pts',(14.2763577914438,18.8079605728532,72.37988723703));
#44789=CARTESIAN_POINT('Ctrl Pts',(14.2832727198514,18.9055511860275,72.3860389693211));
#44790=CARTESIAN_POINT('Ctrl Pts',(14.2832727198514,19.0944488139725,72.3860389693211));
#44791=CARTESIAN_POINT('Ctrl Pts',(14.2763577914438,19.1920394271468,72.37988723703));
#44792=CARTESIAN_POINT('Ctrl Pts',(14.2471849704709,19.3860037650969,72.354242145795));
#44793=CARTESIAN_POINT('Ctrl Pts',(14.2249320231436,19.4823795011934,72.3347583749636));
#44794=CARTESIAN_POINT('Ctrl Pts',(14.1362038196909,19.7594380075451,72.2585860295575));
#44795=CARTESIAN_POINT('Ctrl Pts',(14.0464667888171,19.9277656902715,72.1833081799824));
#44796=CARTESIAN_POINT('Ctrl Pts',(13.8352776378501,20.193547206592,72.0175354868236));
#44797=CARTESIAN_POINT('Ctrl Pts',(13.699571421043,20.3089065123171,71.9159238588941));
#44798=CARTESIAN_POINT('Ctrl Pts',(13.4702718108381,20.4238367380946,71.7589489349143));
#44799=CARTESIAN_POINT('Ctrl Pts',(13.3896280268035,20.4528504393822,71.7058714058911));
#44800=CARTESIAN_POINT('Ctrl Pts',(13.2253894088528,20.4909365811355,71.6024109718344));
#44801=CARTESIAN_POINT('Ctrl Pts',(13.1417904888991,20.5,71.5520312323997));
#44802=CARTESIAN_POINT('Ctrl Pts',(12.9782095111009,20.5,71.4575877108337));
#44803=CARTESIAN_POINT('Ctrl Pts',(12.8927799169376,20.4909365811355,71.4103787921422));
#44804=CARTESIAN_POINT('Ctrl Pts',(12.7210612437826,20.4528504393822,71.3198741937427));
#44805=CARTESIAN_POINT('Ctrl Pts',(12.6347728632611,20.4238367380946,71.2765733926231));
#44806=CARTESIAN_POINT('Ctrl Pts',(12.384178786235,20.3089065123171,71.1564815670977));
#44807=CARTESIAN_POINT('Ctrl Pts',(12.2283274267246,20.193547206592,71.0897623498559));
#44808=CARTESIAN_POINT('Ctrl Pts',(11.9791694877118,19.9277656902715,70.9897535266942));
#44809=CARTESIAN_POINT('Ctrl Pts',(11.8691084422006,19.7594380075451,70.9496779030849));
#44810=CARTESIAN_POINT('Ctrl Pts',(11.7587771542868,19.4823795011934,70.9109231975657));
#44811=CARTESIAN_POINT('Ctrl Pts',(11.7307772401216,19.3860037650969,70.901393465287));
#44812=CARTESIAN_POINT('Ctrl Pts',(11.6939815291433,19.1920394271468,70.8889516068419));
#44813=CARTESIAN_POINT('Ctrl Pts',(11.6851965084981,19.0944488139725,70.8860389693211));
#44814=CARTESIAN_POINT('Ctrl Pts',(11.6851965084981,19.,70.8860389693211));
#44815=CARTESIAN_POINT('Ctrl Pts',(9.30967733958527,14.8450000545077,81.0024999826628));
#44816=CARTESIAN_POINT('Ctrl Pts',(9.49399963863882,14.8449377785778,81.0025197906594));
#44817=CARTESIAN_POINT('Ctrl Pts',(9.8599726667903,14.9548208468277,80.9647069817074));
#44818=CARTESIAN_POINT('Ctrl Pts',(10.1635903263261,15.313863273745,80.8797718802955));
#44819=CARTESIAN_POINT('Ctrl Pts',(10.2636542832646,15.6732395795295,80.8470492838448));
#44820=CARTESIAN_POINT('Ctrl Pts',(10.2585828488274,16.0491061870486,80.8485595236358));
#44821=CARTESIAN_POINT('Ctrl Pts',(10.1358339345559,16.3074452995727,80.8893379358817));
#44822=CARTESIAN_POINT('Ctrl Pts',(9.99531238077664,16.4635283817546,80.9233309936752));
#44823=CARTESIAN_POINT('Ctrl Pts',(9.97541394843821,16.4837399726203,80.927922801608));
#44824=CARTESIAN_POINT('Ctrl Pts',(9.8715454189663,16.5803680094737,80.9507853431027));
#44825=CARTESIAN_POINT('Ctrl Pts',(9.66533594109898,16.7118893446204,80.988220546323));
#44826=CARTESIAN_POINT('Ctrl Pts',(9.39513127992021,16.760496532074,81.0043748388839));
#44827=CARTESIAN_POINT('Ctrl Pts',(9.22386882135598,16.7525596923286,81.0017749459923));
#44828=CARTESIAN_POINT('Ctrl Pts',(9.10596245168451,16.7364763479619,80.9967260931912));
#44829=CARTESIAN_POINT('Ctrl Pts',(8.90305460225939,16.6788818244957,80.9788324346323));
#44830=CARTESIAN_POINT('Ctrl Pts',(8.74872208287691,16.5802588408379,80.9509216345009));
#44831=CARTESIAN_POINT('Ctrl Pts',(8.52753199996129,16.3746224120349,80.9025147999549));
#44832=CARTESIAN_POINT('Ctrl Pts',(8.32895235429463,16.0324014611137,80.8376717466604));
#44833=CARTESIAN_POINT('Ctrl Pts',(8.37228193702135,15.425412033927,80.8539764039352));
#44834=CARTESIAN_POINT('Ctrl Pts',(8.67833944769248,15.0414439730474,80.9436419813148));
#44835=CARTESIAN_POINT('Ctrl Pts',(9.02217645440192,14.8743106493543,80.9926787754169));
#44836=CARTESIAN_POINT('Ctrl Pts',(9.21392517477995,14.8450324057486,81.00248969276));
#44837=CARTESIAN_POINT('Ctrl Pts',(9.30967733958527,14.8450000545077,81.0024999826628));
#44838=CARTESIAN_POINT('Ctrl Pts',(9.30968970356266,14.8950000532224,81.0524999841305));
#44839=CARTESIAN_POINT('Ctrl Pts',(9.48694528401203,14.8947370356301,81.0524949998533));
#44840=CARTESIAN_POINT('Ctrl Pts',(9.83862077660686,15.0031144336227,81.0177967437848));
#44841=CARTESIAN_POINT('Ctrl Pts',(10.1232202750603,15.3462669734862,80.9409650825406));
#44842=CARTESIAN_POINT('Ctrl Pts',(10.2153941656315,15.6820641892916,80.9118514108146));
#44843=CARTESIAN_POINT('Ctrl Pts',(10.2108309919214,16.0317404696965,80.9131375839316));
#44844=CARTESIAN_POINT('Ctrl Pts',(10.0973923997464,16.2744031824593,80.9496392785122));
#44845=CARTESIAN_POINT('Ctrl Pts',(9.96503976415596,16.4235992138869,80.9803887350985));
#44846=CARTESIAN_POINT('Ctrl Pts',(9.94625219275646,16.4428812429394,80.984549686419));
#44847=CARTESIAN_POINT('Ctrl Pts',(9.84806730694828,16.5354259082215,81.0052823264233));
#44848=CARTESIAN_POINT('Ctrl Pts',(9.65171070267945,16.6627611502429,81.039406645323));
#44849=CARTESIAN_POINT('Ctrl Pts',(9.39189564693647,16.7104082463205,81.0542222672945));
#44850=CARTESIAN_POINT('Ctrl Pts',(9.22714789308243,16.7026045728515,81.0518450119684));
#44851=CARTESIAN_POINT('Ctrl Pts',(9.11386983193031,16.6869539104283,81.0472385997827));
#44852=CARTESIAN_POINT('Ctrl Pts',(8.91905457715012,16.6307128161155,81.0308207592159));
#44853=CARTESIAN_POINT('Ctrl Pts',(8.77233148999154,16.5354389845187,81.0054772661211));
#44854=CARTESIAN_POINT('Ctrl Pts',(8.56280532687061,16.3380842628862,80.9614017072328));
#44855=CARTESIAN_POINT('Ctrl Pts',(8.37950980214853,16.0152517876383,80.9035554548782));
#44856=CARTESIAN_POINT('Ctrl Pts',(8.41869689342038,15.4524118992523,80.9178658102062));
#44857=CARTESIAN_POINT('Ctrl Pts',(8.7042245777961,15.0861817681023,80.9985551299171));
#44858=CARTESIAN_POINT('Ctrl Pts',(9.03346590578496,14.9235641805984,81.0436043674832));
#44859=CARTESIAN_POINT('Ctrl Pts',(9.21745201882799,14.895086151504,81.0524111931971));
#44860=CARTESIAN_POINT('Ctrl Pts',(9.30968970356266,14.8950000532224,81.0524999841305));
#44861=CARTESIAN_POINT('Ctrl Pts',(9.30970206754004,14.9450000519371,81.1024999855982));
#44862=CARTESIAN_POINT('Ctrl Pts',(9.47990202593708,14.9451429231465,81.102539555259));
#44863=CARTESIAN_POINT('Ctrl Pts',(9.81719222545616,15.0510938587472,81.0708839943767));
#44864=CARTESIAN_POINT('Ctrl Pts',(10.082929561504,15.3789703241095,81.0021370479354));
#44865=CARTESIAN_POINT('Ctrl Pts',(10.1671718631524,15.6910626190305,80.9766251480691));
#44866=CARTESIAN_POINT('Ctrl Pts',(10.1629882783727,16.0143158338321,80.9777373292404));
#44867=CARTESIAN_POINT('Ctrl Pts',(10.0589372173338,16.2419140185898,81.0098891375199));
#44868=CARTESIAN_POINT('Ctrl Pts',(9.93468300206258,16.3835400150001,81.0374294022131));
#44869=CARTESIAN_POINT('Ctrl Pts',(9.91702810156538,16.4020006342589,81.0411540570315));
#44870=CARTESIAN_POINT('Ctrl Pts',(9.82447906807606,16.4904948345281,81.0597504804512));
#44871=CARTESIAN_POINT('Ctrl Pts',(9.6380201680922,16.613611387635,81.0905702398648));
#44872=CARTESIAN_POINT('Ctrl Pts',(9.3884855334551,16.6602375621895,81.1040231423092));
#44873=CARTESIAN_POINT('Ctrl Pts',(9.23037903157421,16.6526560365432,81.1018484321131));
#44874=CARTESIAN_POINT('Ctrl Pts',(9.12160324597793,16.6373382197703,81.0976495064985));
#44875=CARTESIAN_POINT('Ctrl Pts',(8.93517297178808,16.5827079559131,81.0828394981346));
#44876=CARTESIAN_POINT('Ctrl Pts',(8.79555624957257,16.4904071185435,81.0598179414916));
#44877=CARTESIAN_POINT('Ctrl Pts',(8.5984073178612,16.3020445325207,81.0204404594761));
#44878=CARTESIAN_POINT('Ctrl Pts',(8.42959604077383,15.9978112453145,80.969179699637));
#44879=CARTESIAN_POINT('Ctrl Pts',(8.4652692759342,15.479755280664,80.9818504274788));
#44880=CARTESIAN_POINT('Ctrl Pts',(8.73064802942305,15.1307315854457,81.0537405736822));
#44881=CARTESIAN_POINT('Ctrl Pts',(9.04447343955803,14.9729914718726,81.0943901114622));
#44882=CARTESIAN_POINT('Ctrl Pts',(9.22144276309338,14.9449763675702,81.1025708100384));
#44883=CARTESIAN_POINT('Ctrl Pts',(9.30970206754004,14.9450000519371,81.1024999855982));
#44884=CARTESIAN_POINT('Ctrl Pts',(9.30971443151743,14.9950000506518,81.1524999870659));
#44885=CARTESIAN_POINT('Ctrl Pts',(9.47284767131029,14.9949421801988,81.1525147644529));
#44886=CARTESIAN_POINT('Ctrl Pts',(9.79584033527272,15.0993874455422,81.1239737564541));
#44887=CARTESIAN_POINT('Ctrl Pts',(10.0425595102383,15.4113740238506,81.0633302501805));
#44888=CARTESIAN_POINT('Ctrl Pts',(10.1189117455193,15.6998872287926,81.0414272750389));
#44889=CARTESIAN_POINT('Ctrl Pts',(10.1152364214667,15.99695011648,81.0423153895362));
#44890=CARTESIAN_POINT('Ctrl Pts',(10.0204956825243,16.2088719014764,81.0701904801504));
#44891=CARTESIAN_POINT('Ctrl Pts',(9.9044103854419,16.3436108471324,81.0944871436364));
#44892=CARTESIAN_POINT('Ctrl Pts',(9.88786634588363,16.361141904578,81.0977809418426));
#44893=CARTESIAN_POINT('Ctrl Pts',(9.80100095605804,16.4455527332759,81.1142474637718));
#44894=CARTESIAN_POINT('Ctrl Pts',(9.62439492967267,16.5644831932575,81.1417563388649));
#44895=CARTESIAN_POINT('Ctrl Pts',(9.38524990047136,16.6101492764359,81.1538705707198));
#44896=CARTESIAN_POINT('Ctrl Pts',(9.23365810330067,16.6027009170661,81.1519184980892));
#44897=CARTESIAN_POINT('Ctrl Pts',(9.12951062622373,16.5878157822367,81.1481620130899));
#44898=CARTESIAN_POINT('Ctrl Pts',(8.9511729466788,16.5345389475329,81.1348278227182));
#44899=CARTESIAN_POINT('Ctrl Pts',(8.8191656566872,16.4455872622242,81.1143735731117));
#44900=CARTESIAN_POINT('Ctrl Pts',(8.63368064477052,16.265506383372,81.0793273667541));
#44901=CARTESIAN_POINT('Ctrl Pts',(8.48015348862773,15.9806615718392,81.0350634078547));
#44902=CARTESIAN_POINT('Ctrl Pts',(8.51168423233323,15.5067551459893,81.0457398337499));
#44903=CARTESIAN_POINT('Ctrl Pts',(8.75653315952666,15.1754693805007,81.1086537222845));
#44904=CARTESIAN_POINT('Ctrl Pts',(9.05576289094108,15.0222450031167,81.1453157035286));
#44905=CARTESIAN_POINT('Ctrl Pts',(9.22496960714143,14.9950301133256,81.1524923104755));
#44906=CARTESIAN_POINT('Ctrl Pts',(9.30971443151743,14.9950000506518,81.1524999870659));
#44907=CARTESIAN_POINT('',(9.30967733958527,14.8450000545077,81.0024999826628));
#44908=CARTESIAN_POINT('',(9.30967733958527,14.8450000545077,81.0024999826628));
#44909=CARTESIAN_POINT('',(8.76439716203066,16.5827816051055,80.9526008949626));
#44910=CARTESIAN_POINT('Ctrl Pts',(9.30967733958527,14.8450000545077,81.0024999826628));
#44911=CARTESIAN_POINT('Ctrl Pts',(9.21392517477995,14.8450324057486,81.00248969276));
#44912=CARTESIAN_POINT('Ctrl Pts',(9.02217645440192,14.8743106493543,80.9926787754169));
#44913=CARTESIAN_POINT('Ctrl Pts',(8.67833944769248,15.0414439730474,80.9436419813148));
#44914=CARTESIAN_POINT('Ctrl Pts',(8.37228193702135,15.425412033927,80.8539764039352));
#44915=CARTESIAN_POINT('Ctrl Pts',(8.32895235429463,16.0324014611137,80.8376717466604));
#44916=CARTESIAN_POINT('Ctrl Pts',(8.52753199996129,16.3746224120349,80.9025147999549));
#44917=CARTESIAN_POINT('Ctrl Pts',(8.69606757651563,16.5313068964027,80.9393983422089));
#44918=CARTESIAN_POINT('Ctrl Pts',(8.72917682559677,16.5580725998915,80.9461192566062));
#44919=CARTESIAN_POINT('Ctrl Pts',(8.76439716203066,16.5827816051055,80.9526008949626));
#44920=CARTESIAN_POINT('',(9.8558137849654,16.5828640996264,80.9524659608699));
#44921=CARTESIAN_POINT('Ctrl Pts',(8.76439716203066,16.5827816051055,80.9526008949626));
#44922=CARTESIAN_POINT('Ctrl Pts',(8.82529403548109,16.6255041147677,80.9638078154724));
#44923=CARTESIAN_POINT('Ctrl Pts',(8.94554131631809,16.6909414961979,80.9825791736412));
#44924=CARTESIAN_POINT('Ctrl Pts',(9.10596245168451,16.7364763479619,80.9967260931912));
#44925=CARTESIAN_POINT('Ctrl Pts',(9.22386882135598,16.7525596923286,81.0017749459923));
#44926=CARTESIAN_POINT('Ctrl Pts',(9.39513127992021,16.760496532074,81.0043748388839));
#44927=CARTESIAN_POINT('Ctrl Pts',(9.62133087647619,16.7198054272509,80.9908514065198));
#44928=CARTESIAN_POINT('Ctrl Pts',(9.79484346501603,16.6255969681486,80.9637281582169));
#44929=CARTESIAN_POINT('Ctrl Pts',(9.8558137849654,16.5828640996264,80.9524659608699));
#44930=CARTESIAN_POINT('Ctrl Pts',(9.8558137849654,16.5828640996264,80.9524659608699));
#44931=CARTESIAN_POINT('Ctrl Pts',(9.8910765999414,16.5581491032586,80.9459523525831));
#44932=CARTESIAN_POINT('Ctrl Pts',(9.92422356777855,16.5313619618221,80.9391903357486));
#44933=CARTESIAN_POINT('Ctrl Pts',(9.97541394843821,16.4837399726203,80.927922801608));
#44934=CARTESIAN_POINT('Ctrl Pts',(9.99531238077664,16.4635283817546,80.9233309936752));
#44935=CARTESIAN_POINT('Ctrl Pts',(10.1358339345559,16.3074452995727,80.8893379358817));
#44936=CARTESIAN_POINT('Ctrl Pts',(10.2585828488274,16.0491061870486,80.8485595236358));
#44937=CARTESIAN_POINT('Ctrl Pts',(10.2636542832646,15.6732395795295,80.8470492838448));
#44938=CARTESIAN_POINT('Ctrl Pts',(10.1635903263261,15.313863273745,80.8797718802955));
#44939=CARTESIAN_POINT('Ctrl Pts',(9.8599726667903,14.9548208468277,80.9647069817074));
#44940=CARTESIAN_POINT('Ctrl Pts',(9.49399963863882,14.8449377785778,81.0025197906594));
#44941=CARTESIAN_POINT('Ctrl Pts',(9.30967733958527,14.8450000545077,81.0024999826628));
#44942=CARTESIAN_POINT('Origin',(9.31,18.775,78.));
#44943=CARTESIAN_POINT('',(6.3075,14.15,78.));
#44944=CARTESIAN_POINT('Origin',(9.31,14.15,78.));
#44945=CARTESIAN_POINT('',(6.3075,23.4,78.));
#44946=CARTESIAN_POINT('',(6.3075,18.775,78.));
#44947=CARTESIAN_POINT('Origin',(9.31,23.4,78.));
#44948=CARTESIAN_POINT('Origin',(9.31,19.,78.));
#44949=CARTESIAN_POINT('',(9.31,19.,97.2));
#44950=CARTESIAN_POINT('Origin',(9.31,19.,99.));
#44951=CARTESIAN_POINT('',(1.0383798211071,19.,95.3268664107545));
#44952=CARTESIAN_POINT('Origin',(9.31,19.,78.));
#44953=CARTESIAN_POINT('',(-1.55969639024622,19.,93.8268664107545));
#44954=CARTESIAN_POINT('Ctrl Pts',(-1.55969639024622,19.,93.8268664107545));
#44955=CARTESIAN_POINT('Ctrl Pts',(-1.55969639024622,19.1298398798308,93.8268664107545));
#44956=CARTESIAN_POINT('Ctrl Pts',(-1.55286934050649,19.2576342464927,93.8486597278194));
#44957=CARTESIAN_POINT('Ctrl Pts',(-1.52254836481685,19.5361665210634,93.9423766588895));
#44958=CARTESIAN_POINT('Ctrl Pts',(-1.49582215684855,19.6785504797858,94.0239193323177));
#44959=CARTESIAN_POINT('Ctrl Pts',(-1.41151331058044,19.9800578502247,94.2616163590086));
#44960=CARTESIAN_POINT('Ctrl Pts',(-1.34726058145713,20.1214477955687,94.4315221156896));
#44961=CARTESIAN_POINT('Ctrl Pts',(-1.18695676759168,20.3384257002779,94.7741079267736));
#44962=CARTESIAN_POINT('Ctrl Pts',(-1.08872043557327,20.4154002764241,94.9509005045226));
#44963=CARTESIAN_POINT('Ctrl Pts',(-0.91501820464108,20.4756548309858,95.1525146204047));
#44964=CARTESIAN_POINT('Ctrl Pts',(-0.860662478856494,20.4878793574952,
95.20581219399));
#44965=CARTESIAN_POINT('Ctrl Pts',(-0.758171101748774,20.4989413461778,
95.2849671751815));
#44966=CARTESIAN_POINT('Ctrl Pts',(-0.714349205355399,20.5007261344951,
95.3135640992347));
#44967=CARTESIAN_POINT('Ctrl Pts',(-0.617576626276311,20.4986621094877,
95.3656661602697));
#44968=CARTESIAN_POINT('Ctrl Pts',(-0.5654286151719,20.4943583996059,95.3878690863923));
#44969=CARTESIAN_POINT('Ctrl Pts',(-0.413657365059915,20.4735716734213,
95.4385197926724));
#44970=CARTESIAN_POINT('Ctrl Pts',(-0.31263191661929,20.4502685845107,95.4563416379516));
#44971=CARTESIAN_POINT('Ctrl Pts',(-0.0789744689677987,20.3775229034925,
95.4774958870508));
#44972=CARTESIAN_POINT('Ctrl Pts',(0.061044700769779,20.3188989837733,95.4741371363919));
#44973=CARTESIAN_POINT('Ctrl Pts',(0.393973711379464,20.1330764472051,95.4477411901324));
#44974=CARTESIAN_POINT('Ctrl Pts',(0.58454770192275,19.9855206415407,95.4165926999351));
#44975=CARTESIAN_POINT('Ctrl Pts',(0.847937571353683,19.6626095831238,95.3677669972487));
#44976=CARTESIAN_POINT('Ctrl Pts',(0.936366028690045,19.5066066529301,95.3489694894714));
#44977=CARTESIAN_POINT('Ctrl Pts',(1.02128074726238,19.2262024684657,95.3306789801616));
#44978=CARTESIAN_POINT('Ctrl Pts',(1.03837982110709,19.1137113861875,95.3268664107545));
#44979=CARTESIAN_POINT('Ctrl Pts',(1.03837982110709,19.,95.3268664107545));
#44980=CARTESIAN_POINT('',(-9.83131656913913,19.,79.5));
#44981=CARTESIAN_POINT('Origin',(9.31,19.,78.));
#44982=CARTESIAN_POINT('',(-9.83131656913913,19.,76.5));
#44983=CARTESIAN_POINT('Ctrl Pts',(-9.83131656913913,19.,76.5));
#44984=CARTESIAN_POINT('Ctrl Pts',(-9.83131656913913,19.1245217970218,76.5));
#44985=CARTESIAN_POINT('Ctrl Pts',(-9.84554380418068,19.2486348123039,76.5154677646786));
#44986=CARTESIAN_POINT('Ctrl Pts',(-9.90682498456632,19.5152363108006,76.5833051354963));
#44987=CARTESIAN_POINT('Ctrl Pts',(-9.95871278232153,19.6513770277057,76.6411156315615));
#44988=CARTESIAN_POINT('Ctrl Pts',(-10.1026555664131,19.9291519129669,76.8087481691482));
#44989=CARTESIAN_POINT('Ctrl Pts',(-10.2014133131777,20.0630977664656,76.9273940576885));
#44990=CARTESIAN_POINT('Ctrl Pts',(-10.4149894821051,20.2954859145557,77.2185345135431));
#44991=CARTESIAN_POINT('Ctrl Pts',(-10.5280386633462,20.3847092201747,77.3927468017688));
#44992=CARTESIAN_POINT('Ctrl Pts',(-10.6573116577679,20.4769000895387,77.7049195202664));
#44993=CARTESIAN_POINT('Ctrl Pts',(-10.6848483892464,20.4935592903711,77.8229433494293));
#44994=CARTESIAN_POINT('Ctrl Pts',(-10.7001274699635,20.5032447555465,78.0385628545257));
#44995=CARTESIAN_POINT('Ctrl Pts',(-10.6896585844537,20.4969058005831,78.1429558632871));
#44996=CARTESIAN_POINT('Ctrl Pts',(-10.6331076337369,20.4596343864514,78.3660543960096));
#44997=CARTESIAN_POINT('Ctrl Pts',(-10.5835751290906,20.4257618686536,78.4798599905703));
#44998=CARTESIAN_POINT('Ctrl Pts',(-10.4408937377185,20.3131243051215,78.7457519131079));
#44999=CARTESIAN_POINT('Ctrl Pts',(-10.3291283199371,20.2132427857327,78.9037637004356));
#45000=CARTESIAN_POINT('Ctrl Pts',(-10.1184813956406,19.9505788790836,79.1742528903653));
#45001=CARTESIAN_POINT('Ctrl Pts',(-10.0216936341199,19.7964852740788,79.2865908485361));
#45002=CARTESIAN_POINT('Ctrl Pts',(-9.89489746957705,19.4764502513109,79.4303757672511));
#45003=CARTESIAN_POINT('Ctrl Pts',(-9.85522800261023,19.3240506827592,79.4737983676688));
#45004=CARTESIAN_POINT('Ctrl Pts',(-9.83395109612093,19.1071959085279,79.4971214837868));
#45005=CARTESIAN_POINT('Ctrl Pts',(-9.83131656913913,19.0536635113807,79.5));
#45006=CARTESIAN_POINT('Ctrl Pts',(-9.83131656913913,19.,79.5));
#45007=CARTESIAN_POINT('',(-1.55969639024623,19.,62.1731335892455));
#45008=CARTESIAN_POINT('Origin',(9.31,19.,78.));
#45009=CARTESIAN_POINT('',(1.03837982110709,19.,60.6731335892455));
#45010=CARTESIAN_POINT('Ctrl Pts',(1.03837982110709,19.,60.6731335892455));
#45011=CARTESIAN_POINT('Ctrl Pts',(1.03837982110709,19.1298398798308,60.6731335892455));
#45012=CARTESIAN_POINT('Ctrl Pts',(1.01609273002626,19.2576342464927,60.6681493292206));
#45013=CARTESIAN_POINT('Ctrl Pts',(0.919770999110034,19.5361665210635,60.6475495989003));
#45014=CARTESIAN_POINT('Ctrl Pts',(0.835789868444578,19.6785504797858,60.6299238372336));
#45015=CARTESIAN_POINT('Ctrl Pts',(0.587783781791739,19.9800578502252,60.58408892652));
#45016=CARTESIAN_POINT('Ctrl Pts',(0.408514715694908,20.1214477955691,60.5547805438627));
#45017=CARTESIAN_POINT('Ctrl Pts',(0.0316747933878957,20.338425700278,60.5223148134518));
#45018=CARTESIAN_POINT('Ctrl Pts',(-0.170550236152408,20.4154002764241,
60.5189936836799));
#45019=CARTESIAN_POINT('Ctrl Pts',(-0.432004297734002,20.4756548309859,
60.5686171704201));
#45020=CARTESIAN_POINT('Ctrl Pts',(-0.505339213311197,20.4878793574952,
60.5890418229981));
#45021=CARTESIAN_POINT('Ctrl Pts',(-0.625135126412895,20.4989413461778,
60.6382244686464));
#45022=CARTESIAN_POINT('Ctrl Pts',(-0.671811737309813,20.5007261344951,
60.6618768821385));
#45023=CARTESIAN_POINT('Ctrl Pts',(-0.765319735295206,20.4986621094877,
60.7196333634933));
#45024=CARTESIAN_POINT('Ctrl Pts',(-0.810622038907963,20.4943583996059,
60.7536934028052));
#45025=CARTESIAN_POINT('Ctrl Pts',(-0.930372462322086,20.4735716734213,
60.8598058078263));
#45026=CARTESIAN_POINT('Ctrl Pts',(-0.996319357296532,20.4502685845106,
60.9383854899651));
#45027=CARTESIAN_POINT('Ctrl Pts',(-1.13146819824008,20.3775229034925,61.1301616508649));
#45028=CARTESIAN_POINT('Ctrl Pts',(-1.19856901971327,20.3188989837734,61.2531011842039));
#45029=CARTESIAN_POINT('Ctrl Pts',(-1.3421739650006,20.133076447205,61.5546241381787));
#45030=CARTESIAN_POINT('Ctrl Pts',(-1.41048557647178,19.9855206415405,61.7352403003884));
#45031=CARTESIAN_POINT('Ctrl Pts',(-1.49989621230313,19.6626095831239,61.9877554697581));
#45032=CARTESIAN_POINT('Ctrl Pts',(-1.52783132170843,19.5066066529302,62.0737355141175));
#45033=CARTESIAN_POINT('Ctrl Pts',(-1.55444863528416,19.2262024684657,62.1564190722112));
#45034=CARTESIAN_POINT('Ctrl Pts',(-1.55969639024623,19.1137113861875,62.1731335892455));
#45035=CARTESIAN_POINT('Ctrl Pts',(-1.55969639024623,19.,62.1731335892455));
#45036=CARTESIAN_POINT('',(17.5816201788929,19.,60.6731335892455));
#45037=CARTESIAN_POINT('Origin',(9.31,19.,78.));
#45038=CARTESIAN_POINT('',(20.1796963902462,19.,62.1731335892455));
#45039=CARTESIAN_POINT('Ctrl Pts',(20.1796963902462,19.,62.1731335892455));
#45040=CARTESIAN_POINT('Ctrl Pts',(20.1796963902462,19.1298398798308,62.1731335892455));
#45041=CARTESIAN_POINT('Ctrl Pts',(20.1728693405065,19.2576342464928,62.1513402721806));
#45042=CARTESIAN_POINT('Ctrl Pts',(20.1425483648168,19.5361665210635,62.0576233411105));
#45043=CARTESIAN_POINT('Ctrl Pts',(20.1158221568485,19.6785504797858,61.9760806676823));
#45044=CARTESIAN_POINT('Ctrl Pts',(20.0315133105802,19.9800578502254,61.7383836409908));
#45045=CARTESIAN_POINT('Ctrl Pts',(19.9672605814568,20.1214477955692,61.5684778843096));
#45046=CARTESIAN_POINT('Ctrl Pts',(19.8069567675917,20.3384257002779,61.2258920732264));
#45047=CARTESIAN_POINT('Ctrl Pts',(19.7087204355733,20.4154002764241,61.0490994954775));
#45048=CARTESIAN_POINT('Ctrl Pts',(19.535018204641,20.4756548309859,60.8474853795952));
#45049=CARTESIAN_POINT('Ctrl Pts',(19.4806624788565,20.4878793574952,60.79418780601));
#45050=CARTESIAN_POINT('Ctrl Pts',(19.3781711017488,20.4989413461778,60.7150328248185));
#45051=CARTESIAN_POINT('Ctrl Pts',(19.3343492053554,20.5007261344951,60.6864359007653));
#45052=CARTESIAN_POINT('Ctrl Pts',(19.2375766262763,20.4986621094877,60.6343338397303));
#45053=CARTESIAN_POINT('Ctrl Pts',(19.1854286151718,20.4943583996059,60.6121309136077));
#45054=CARTESIAN_POINT('Ctrl Pts',(19.0336573650599,20.4735716734213,60.5614802073276));
#45055=CARTESIAN_POINT('Ctrl Pts',(18.9326319166192,20.4502685845106,60.5436583620484));
#45056=CARTESIAN_POINT('Ctrl Pts',(18.6989744689681,20.3775229034925,60.5225041129492));
#45057=CARTESIAN_POINT('Ctrl Pts',(18.5589552992305,20.3188989837735,60.5258628636081));
#45058=CARTESIAN_POINT('Ctrl Pts',(18.2260262886202,20.1330764472049,60.5522588098677));
#45059=CARTESIAN_POINT('Ctrl Pts',(18.035452298077,19.9855206415404,60.583407300065));
#45060=CARTESIAN_POINT('Ctrl Pts',(17.7720624286463,19.6626095831238,60.6322330027514));
#45061=CARTESIAN_POINT('Ctrl Pts',(17.68363397131,19.5066066529301,60.6510305105286));
#45062=CARTESIAN_POINT('Ctrl Pts',(17.5987192527376,19.2262024684657,60.6693210198384));
#45063=CARTESIAN_POINT('Ctrl Pts',(17.5816201788929,19.1137113861875,60.6731335892455));
#45064=CARTESIAN_POINT('Ctrl Pts',(17.5816201788929,19.,60.6731335892455));
#45065=CARTESIAN_POINT('',(28.4513165691391,19.,76.5));
#45066=CARTESIAN_POINT('Origin',(9.31,19.,78.));
#45067=CARTESIAN_POINT('',(28.4513165691391,19.,79.5));
#45068=CARTESIAN_POINT('Ctrl Pts',(28.4513165691391,19.,79.5));
#45069=CARTESIAN_POINT('Ctrl Pts',(28.4513165691391,19.1245217970218,79.5));
#45070=CARTESIAN_POINT('Ctrl Pts',(28.4655438041807,19.248634812304,79.4845322353214));
#45071=CARTESIAN_POINT('Ctrl Pts',(28.5268249845663,19.5152363108006,79.4166948645036));
#45072=CARTESIAN_POINT('Ctrl Pts',(28.5787127823215,19.6513770277057,79.3588843684386));
#45073=CARTESIAN_POINT('Ctrl Pts',(28.7226555664131,19.9291519129669,79.1912518308518));
#45074=CARTESIAN_POINT('Ctrl Pts',(28.8214133131777,20.0630977664656,79.0726059423115));
#45075=CARTESIAN_POINT('Ctrl Pts',(29.0349894821052,20.2954859145559,78.7814654864567));
#45076=CARTESIAN_POINT('Ctrl Pts',(29.1480386633463,20.3847092201747,78.607253198231));
#45077=CARTESIAN_POINT('Ctrl Pts',(29.2773116577678,20.4769000895386,78.2950804797337));
#45078=CARTESIAN_POINT('Ctrl Pts',(29.3048483892464,20.4935592903711,78.1770566505708));
#45079=CARTESIAN_POINT('Ctrl Pts',(29.3201274699635,20.5032447555465,77.9614371454743));
#45080=CARTESIAN_POINT('Ctrl Pts',(29.3096585844537,20.4969058005831,77.8570441367129));
#45081=CARTESIAN_POINT('Ctrl Pts',(29.2531076337369,20.4596343864514,77.6339456039904));
#45082=CARTESIAN_POINT('Ctrl Pts',(29.2035751290906,20.4257618686536,77.5201400094297));
#45083=CARTESIAN_POINT('Ctrl Pts',(29.0608937377183,20.3131243051213,77.2542480868917));
#45084=CARTESIAN_POINT('Ctrl Pts',(28.9491283199369,20.2132427857324,77.0962362995642));
#45085=CARTESIAN_POINT('Ctrl Pts',(28.7384813956406,19.9505788790835,76.8257471096347));
#45086=CARTESIAN_POINT('Ctrl Pts',(28.6416936341199,19.7964852740788,76.7134091514639));
#45087=CARTESIAN_POINT('Ctrl Pts',(28.5148974695771,19.4764502513109,76.5696242327489));
#45088=CARTESIAN_POINT('Ctrl Pts',(28.4752280026102,19.3240506827592,76.5262016323312));
#45089=CARTESIAN_POINT('Ctrl Pts',(28.4539510961209,19.1071959085279,76.5028785162132));
#45090=CARTESIAN_POINT('Ctrl Pts',(28.4513165691391,19.0536635113807,76.5));
#45091=CARTESIAN_POINT('Ctrl Pts',(28.4513165691391,19.,76.5));
#45092=CARTESIAN_POINT('',(20.1796963902462,19.,93.8268664107545));
#45093=CARTESIAN_POINT('Origin',(9.31,19.,78.));
#45094=CARTESIAN_POINT('',(17.5816201788929,19.,95.3268664107545));
#45095=CARTESIAN_POINT('Ctrl Pts',(17.5816201788929,19.,95.3268664107545));
#45096=CARTESIAN_POINT('Ctrl Pts',(17.5816201788929,19.1298398798308,95.3268664107545));
#45097=CARTESIAN_POINT('Ctrl Pts',(17.6039072699737,19.2576342464928,95.3318506707794));
#45098=CARTESIAN_POINT('Ctrl Pts',(17.70022900089,19.5361665210636,95.3524504010997));
#45099=CARTESIAN_POINT('Ctrl Pts',(17.7842101315555,19.6785504797859,95.3700761627664));
#45100=CARTESIAN_POINT('Ctrl Pts',(18.0322162182082,19.9800578502251,95.41591107348));
#45101=CARTESIAN_POINT('Ctrl Pts',(18.211485284305,20.121447795569,95.4452194561373));
#45102=CARTESIAN_POINT('Ctrl Pts',(18.5883252066121,20.338425700278,95.4776851865482));
#45103=CARTESIAN_POINT('Ctrl Pts',(18.7905502361524,20.4154002764241,95.4810063163201));
#45104=CARTESIAN_POINT('Ctrl Pts',(19.0520042977342,20.4756548309859,95.4313828295798));
#45105=CARTESIAN_POINT('Ctrl Pts',(19.1253392133113,20.4878793574952,95.4109581770019));
#45106=CARTESIAN_POINT('Ctrl Pts',(19.2451351264128,20.4989413461777,95.3617755313536));
#45107=CARTESIAN_POINT('Ctrl Pts',(19.2918117373098,20.5007261344951,95.3381231178615));
#45108=CARTESIAN_POINT('Ctrl Pts',(19.3853197352953,20.4986621094877,95.2803666365067));
#45109=CARTESIAN_POINT('Ctrl Pts',(19.4306220389081,20.4943583996059,95.2463065971947));
#45110=CARTESIAN_POINT('Ctrl Pts',(19.5503724623221,20.4735716734213,95.1401941921737));
#45111=CARTESIAN_POINT('Ctrl Pts',(19.6163193572965,20.4502685845106,95.0616145100349));
#45112=CARTESIAN_POINT('Ctrl Pts',(19.75146819824,20.3775229034925,94.8698383491352));
#45113=CARTESIAN_POINT('Ctrl Pts',(19.8185690197132,20.3188989837735,94.7468988157962));
#45114=CARTESIAN_POINT('Ctrl Pts',(19.9621739650008,20.1330764472048,94.4453758618209));
#45115=CARTESIAN_POINT('Ctrl Pts',(20.0304855764719,19.9855206415402,94.2647596996113));
#45116=CARTESIAN_POINT('Ctrl Pts',(20.1198962123032,19.6626095831237,94.0122445302418));
#45117=CARTESIAN_POINT('Ctrl Pts',(20.1478313217084,19.50660665293,93.9262644858825));
#45118=CARTESIAN_POINT('Ctrl Pts',(20.1744486352842,19.2262024684656,93.8435809277888));
#45119=CARTESIAN_POINT('Ctrl Pts',(20.1796963902462,19.1137113861874,93.8268664107545));
#45120=CARTESIAN_POINT('Ctrl Pts',(20.1796963902462,19.,93.8268664107545));
#45121=CARTESIAN_POINT('Origin',(9.31,19.,78.));
#45122=CARTESIAN_POINT('',(19.3125062814467,17.5,95.3248490824925));
#45123=CARTESIAN_POINT('Ctrl Pts',(19.3125062814467,17.5,95.3248490824925));
#45124=CARTESIAN_POINT('Ctrl Pts',(19.2653612797053,17.5,95.3520682619388));
#45125=CARTESIAN_POINT('Ctrl Pts',(19.2163882916827,17.502946735144,95.3749120396601));
#45126=CARTESIAN_POINT('Ctrl Pts',(19.0831906327501,17.5181479027027,95.424536757463));
#45127=CARTESIAN_POINT('Ctrl Pts',(18.9982617981722,17.5348232538744,95.4440603634893));
#45128=CARTESIAN_POINT('Ctrl Pts',(18.8009075569721,17.5875127881648,95.4720531545667));
#45129=CARTESIAN_POINT('Ctrl Pts',(18.6875380327356,17.6285240662611,95.4750565548865));
#45130=CARTESIAN_POINT('Ctrl Pts',(18.3942021353586,17.7623087481876,95.4666942719671));
#45131=CARTESIAN_POINT('Ctrl Pts',(18.2058843837797,17.8796864892639,95.4425232119164));
#45132=CARTESIAN_POINT('Ctrl Pts',(17.8971879945484,18.1666272894372,95.3925756323412));
#45133=CARTESIAN_POINT('Ctrl Pts',(17.7745791487004,18.3256026756653,95.3678345274791));
#45134=CARTESIAN_POINT('Ctrl Pts',(17.6273835423512,18.6468724886465,95.3370780178918));
#45135=CARTESIAN_POINT('Ctrl Pts',(17.5890720003775,18.7971695012231,95.3285089232078));
#45136=CARTESIAN_POINT('Ctrl Pts',(17.5819451644934,18.9686255097769,95.3269380887608));
#45137=CARTESIAN_POINT('Ctrl Pts',(17.5816201788929,18.984327656238,95.3268664107545));
#45138=CARTESIAN_POINT('Ctrl Pts',(17.5816201788929,19.,95.3268664107545));
#45139=CARTESIAN_POINT('Ctrl Pts',(20.1796963902462,19.,93.8268664107545));
#45140=CARTESIAN_POINT('Ctrl Pts',(20.1796963902462,18.9648000704088,93.8268664107545));
#45141=CARTESIAN_POINT('Ctrl Pts',(20.1791901743517,18.9294832054732,93.8284669499666));
#45142=CARTESIAN_POINT('Ctrl Pts',(20.1738795413826,18.7461724891623,93.8452165866068));
#45143=CARTESIAN_POINT('Ctrl Pts',(20.1608254414315,18.6040823417908,93.8866376596314));
#45144=CARTESIAN_POINT('Ctrl Pts',(20.1142713209593,18.3102983306061,94.0274111126068));
#45145=CARTESIAN_POINT('Ctrl Pts',(20.0777756307246,18.1669858887453,94.1349945295655));
#45146=CARTESIAN_POINT('Ctrl Pts',(19.9621359407356,17.8610717494632,94.441071667855));
#45147=CARTESIAN_POINT('Ctrl Pts',(19.8731660176324,17.7272792212461,94.6533728241667));
#45148=CARTESIAN_POINT('Ctrl Pts',(19.6971324340933,17.5873420162312,94.9529469331406));
#45149=CARTESIAN_POINT('Ctrl Pts',(19.6195169618968,17.5470806517564,95.0646162294015));
#45150=CARTESIAN_POINT('Ctrl Pts',(19.4787984488119,17.5125581835725,95.2059766108471));
#45151=CARTESIAN_POINT('Ctrl Pts',(19.4302635208502,17.5052303115316,95.2473360103154));
#45152=CARTESIAN_POINT('Ctrl Pts',(19.3561746798665,17.5006516995771,95.2984438337642));
#45153=CARTESIAN_POINT('Ctrl Pts',(19.3346302397217,17.5,95.3120758092269));
#45154=CARTESIAN_POINT('Ctrl Pts',(19.3125062814467,17.5,95.3248490824925));
#45155=CARTESIAN_POINT('',(29.3150125628934,17.5,78.));
#45156=CARTESIAN_POINT('Ctrl Pts',(29.3150125628934,17.5,78.));
#45157=CARTESIAN_POINT('Ctrl Pts',(29.3150125628934,17.5,78.1047390770919));
#45158=CARTESIAN_POINT('Ctrl Pts',(29.2974013907771,17.5108310402064,78.2071426028014));
#45159=CARTESIAN_POINT('Ctrl Pts',(29.226922072288,17.5583420169659,78.4339131995391));
#45160=CARTESIAN_POINT('Ctrl Pts',(29.1673418462476,17.6007431024611,78.5542198710694));
#45161=CARTESIAN_POINT('Ctrl Pts',(29.0020601635,17.7393206831897,78.83476146908));
#45162=CARTESIAN_POINT('Ctrl Pts',(28.8769173400547,17.8614426921814,79.0006494510307));
#45163=CARTESIAN_POINT('Ctrl Pts',(28.6701915527651,18.1597175199196,79.2546083244645));
#45164=CARTESIAN_POINT('Ctrl Pts',(28.5867105343723,18.3173213761021,79.3494913085985));
#45165=CARTESIAN_POINT('Ctrl Pts',(28.4853157633783,18.637591898099,79.4629623925713));
#45166=CARTESIAN_POINT('Ctrl Pts',(28.457609981235,18.7870280562669,79.4931146708418));
#45167=CARTESIAN_POINT('Ctrl Pts',(28.4516322653758,18.9628275273603,79.4996547399714));
#45168=CARTESIAN_POINT('Ctrl Pts',(28.4513165691391,18.9814183151259,79.5));
#45169=CARTESIAN_POINT('Ctrl Pts',(28.4513165691391,19.,79.5));
#45170=CARTESIAN_POINT('Ctrl Pts',(28.4513165691391,19.,76.5));
#45171=CARTESIAN_POINT('Ctrl Pts',(28.4513165691391,18.9077230153478,76.5));
#45172=CARTESIAN_POINT('Ctrl Pts',(28.4591147250101,18.8150583449374,76.5085002722188));
#45173=CARTESIAN_POINT('Ctrl Pts',(28.4993679863007,18.5791911526486,76.5528200938006));
#45174=CARTESIAN_POINT('Ctrl Pts',(28.5423240325381,18.4425366457864,76.6002411233075));
#45175=CARTESIAN_POINT('Ctrl Pts',(28.6668807891092,18.1638733921006,76.742921963351));
#45176=CARTESIAN_POINT('Ctrl Pts',(28.7539057616696,18.0287684620774,76.8450091634613));
#45177=CARTESIAN_POINT('Ctrl Pts',(28.9714335308102,17.7609964409145,77.1256645774523));
#45178=CARTESIAN_POINT('Ctrl Pts',(29.1032005944038,17.650192730897,77.3135344313333));
#45179=CARTESIAN_POINT('Ctrl Pts',(29.2538951387463,17.5385627946699,77.6365203536188));
#45180=CARTESIAN_POINT('Ctrl Pts',(29.292937166705,17.5140590169286,77.7600350329524));
#45181=CARTESIAN_POINT('Ctrl Pts',(29.3126407860379,17.5014920111156,77.9228715529961));
#45182=CARTESIAN_POINT('Ctrl Pts',(29.3150125628934,17.5,77.9613132360328));
#45183=CARTESIAN_POINT('Ctrl Pts',(29.3150125628934,17.5,78.));
#45184=CARTESIAN_POINT('',(19.3125062814467,17.5,60.6751509175075));
#45185=CARTESIAN_POINT('Ctrl Pts',(19.3125062814467,17.5,60.6751509175075));
#45186=CARTESIAN_POINT('Ctrl Pts',(19.359651283188,17.5,60.7023700969538));
#45187=CARTESIAN_POINT('Ctrl Pts',(19.4039210690243,17.502946735144,60.7333600598199));
#45188=CARTESIAN_POINT('Ctrl Pts',(19.5134961647636,17.5181479027027,60.8239002572788));
#45189=CARTESIAN_POINT('Ctrl Pts',(19.5728685208448,17.5348232538744,60.8876889825239));
#45190=CARTESIAN_POINT('Ctrl Pts',(19.6957881096408,17.5875127881649,61.0446063734092));
#45191=CARTESIAN_POINT('Ctrl Pts',(19.7550738927337,17.6285240662612,61.1412855612531));
#45192=CARTESIAN_POINT('Ctrl Pts',(19.8944998919804,17.7623087481876,61.3995030416831));
#45193=CARTESIAN_POINT('Ctrl Pts',(19.9677260157295,17.879686489264,61.5746765285594));
#45194=CARTESIAN_POINT('Ctrl Pts',(20.0788183375755,18.1666272894372,61.8669892334777));
#45195=CARTESIAN_POINT('Ctrl Pts',(20.1186963351712,18.3256026756653,61.9855421611418));
#45196=CARTESIAN_POINT('Ctrl Pts',(20.1656582197115,18.6468724886465,62.1283955503593));
#45197=CARTESIAN_POINT('Ctrl Pts',(20.1773929370146,18.7971695012231,62.1658588663088));
#45198=CARTESIAN_POINT('Ctrl Pts',(20.1795959724204,18.968625509777,62.1728163044565));
#45199=CARTESIAN_POINT('Ctrl Pts',(20.1796963902462,18.984327656238,62.1731335892455));
#45200=CARTESIAN_POINT('Ctrl Pts',(20.1796963902462,19.,62.1731335892455));
#45201=CARTESIAN_POINT('Ctrl Pts',(17.5816201788929,19.,60.6731335892455));
#45202=CARTESIAN_POINT('Ctrl Pts',(17.5816201788929,18.9648000704089,60.6731335892455));
#45203=CARTESIAN_POINT('Ctrl Pts',(17.5832593944576,18.9294832054732,60.6727717154639));
#45204=CARTESIAN_POINT('Ctrl Pts',(17.6004203217768,18.7461724891624,60.6689960402053));
#45205=CARTESIAN_POINT('Ctrl Pts',(17.6428190732436,18.604082341791,60.6595906858741));
#45206=CARTESIAN_POINT('Ctrl Pts',(17.7880095199348,18.3102983306063,60.6295210103662));
#45207=CARTESIAN_POINT('Ctrl Pts',(17.8994273371643,18.1669858887454,60.6073354967588));
#45208=CARTESIAN_POINT('Ctrl Pts',(18.2223177594351,17.8610717494634,60.5544438368303));
#45209=CARTESIAN_POINT('Ctrl Pts',(18.4506609156053,17.7272792212462,60.5253434722546));
#45210=CARTESIAN_POINT('Ctrl Pts',(18.7981164960626,17.5873420162312,60.5280059730316));
#45211=CARTESIAN_POINT('Ctrl Pts',(18.9336326795454,17.5470806517564,60.5393882955501));
#45212=CARTESIAN_POINT('Ctrl Pts',(19.1264136175084,17.5125581835725,60.5905739119415));
#45213=CARTESIAN_POINT('Ctrl Pts',(19.1864993721141,17.5052303115316,60.6119266927931));
#45214=CARTESIAN_POINT('Ctrl Pts',(19.267804466045,17.5006516995771,60.6505355994976));
#45215=CARTESIAN_POINT('Ctrl Pts',(19.2903823231718,17.5,60.6623776442419));
#45216=CARTESIAN_POINT('Ctrl Pts',(19.3125062814467,17.5,60.6751509175075));
#45217=CARTESIAN_POINT('',(-0.692506281446699,17.5,60.6751509175075));
#45218=CARTESIAN_POINT('Ctrl Pts',(-0.692506281446699,17.5,60.6751509175075));
#45219=CARTESIAN_POINT('Ctrl Pts',(-0.645361279705448,17.5,60.6479317380612));
#45220=CARTESIAN_POINT('Ctrl Pts',(-0.596388291682915,17.502946735144,60.6250879603399));
#45221=CARTESIAN_POINT('Ctrl Pts',(-0.463190632750145,17.5181479027027,
60.575463242537));
#45222=CARTESIAN_POINT('Ctrl Pts',(-0.378261798172194,17.5348232538744,
60.5559396365107));
#45223=CARTESIAN_POINT('Ctrl Pts',(-0.180907556972113,17.5875127881648,
60.5279468454333));
#45224=CARTESIAN_POINT('Ctrl Pts',(-0.0675380327356137,17.6285240662611,
60.5249434451136));
#45225=CARTESIAN_POINT('Ctrl Pts',(0.225797864641484,17.7623087481876,60.5333057280329));
#45226=CARTESIAN_POINT('Ctrl Pts',(0.414115616220393,17.879686489264,60.5574767880836));
#45227=CARTESIAN_POINT('Ctrl Pts',(0.72281200545154,18.1666272894371,60.6074243676588));
#45228=CARTESIAN_POINT('Ctrl Pts',(0.845420851299561,18.3256026756652,60.6321654725209));
#45229=CARTESIAN_POINT('Ctrl Pts',(0.992616457648736,18.6468724886464,60.6629219821082));
#45230=CARTESIAN_POINT('Ctrl Pts',(1.03092799962253,18.797169501223,60.6714910767922));
#45231=CARTESIAN_POINT('Ctrl Pts',(1.0380548355066,18.9686255097769,60.6730619112392));
#45232=CARTESIAN_POINT('Ctrl Pts',(1.03837982110709,18.984327656238,60.6731335892455));
#45233=CARTESIAN_POINT('Ctrl Pts',(1.03837982110709,19.,60.6731335892455));
#45234=CARTESIAN_POINT('Ctrl Pts',(-1.55969639024623,19.,62.1731335892455));
#45235=CARTESIAN_POINT('Ctrl Pts',(-1.55969639024623,18.9648000704089,62.1731335892455));
#45236=CARTESIAN_POINT('Ctrl Pts',(-1.55919017435171,18.9294832054733,62.1715330500334));
#45237=CARTESIAN_POINT('Ctrl Pts',(-1.55387954138258,18.7461724891625,62.1547834133932));
#45238=CARTESIAN_POINT('Ctrl Pts',(-1.54082544143153,18.6040823417911,62.1133623403687));
#45239=CARTESIAN_POINT('Ctrl Pts',(-1.49427132095936,18.3102983306063,61.9725888873933));
#45240=CARTESIAN_POINT('Ctrl Pts',(-1.45777563072466,18.1669858887455,61.8650054704346));
#45241=CARTESIAN_POINT('Ctrl Pts',(-1.3421359407357,17.8610717494634,61.5589283321452));
#45242=CARTESIAN_POINT('Ctrl Pts',(-1.25316601763253,17.7272792212462,61.3466271758336));
#45243=CARTESIAN_POINT('Ctrl Pts',(-1.0771324340934,17.5873420162312,61.0470530668595));
#45244=CARTESIAN_POINT('Ctrl Pts',(-0.999516961896896,17.5470806517564,
60.9353837705987));
#45245=CARTESIAN_POINT('Ctrl Pts',(-0.85879844881205,17.5125581835725,60.794023389153));
#45246=CARTESIAN_POINT('Ctrl Pts',(-0.81026352085034,17.5052303115316,60.7526639896847));
#45247=CARTESIAN_POINT('Ctrl Pts',(-0.736174679866266,17.5006516995771,
60.7015561662356));
#45248=CARTESIAN_POINT('Ctrl Pts',(-0.714630239721583,17.5,60.687924190773));
#45249=CARTESIAN_POINT('Ctrl Pts',(-0.6925062814467,17.5,60.6751509175075));
#45250=CARTESIAN_POINT('',(-10.6950125628934,17.5,78.));
#45251=CARTESIAN_POINT('Ctrl Pts',(-10.6950125628934,17.5,78.));
#45252=CARTESIAN_POINT('Ctrl Pts',(-10.6950125628934,17.5,77.8952609229081));
#45253=CARTESIAN_POINT('Ctrl Pts',(-10.6774013907771,17.5108310402064,77.7928573971986));
#45254=CARTESIAN_POINT('Ctrl Pts',(-10.606922072288,17.5583420169659,77.5660868004609));
#45255=CARTESIAN_POINT('Ctrl Pts',(-10.5473418462476,17.6007431024612,77.4457801289306));
#45256=CARTESIAN_POINT('Ctrl Pts',(-10.3820601635002,17.7393206831896,77.1652385309203));
#45257=CARTESIAN_POINT('Ctrl Pts',(-10.2569173400549,17.8614426921811,76.9993505489696));
#45258=CARTESIAN_POINT('Ctrl Pts',(-10.0501915527651,18.1597175199196,76.7453916755355));
#45259=CARTESIAN_POINT('Ctrl Pts',(-9.96671053437231,18.3173213761021,76.6505086914015));
#45260=CARTESIAN_POINT('Ctrl Pts',(-9.86531576337833,18.637591898099,76.5370376074287));
#45261=CARTESIAN_POINT('Ctrl Pts',(-9.83760998123497,18.7870280562669,76.5068853291583));
#45262=CARTESIAN_POINT('Ctrl Pts',(-9.83163226537581,18.9628275273603,76.5003452600286));
#45263=CARTESIAN_POINT('Ctrl Pts',(-9.83131656913913,18.9814183151258,76.5));
#45264=CARTESIAN_POINT('Ctrl Pts',(-9.83131656913913,19.,76.5));
#45265=CARTESIAN_POINT('Ctrl Pts',(-9.83131656913913,19.,79.5));
#45266=CARTESIAN_POINT('Ctrl Pts',(-9.83131656913913,18.9077230153478,79.5));
#45267=CARTESIAN_POINT('Ctrl Pts',(-9.83911472501011,18.8150583449374,79.4914997277812));
#45268=CARTESIAN_POINT('Ctrl Pts',(-9.87936798630065,18.5791911526486,79.4471799061994));
#45269=CARTESIAN_POINT('Ctrl Pts',(-9.92232403253812,18.4425366457864,79.3997588766925));
#45270=CARTESIAN_POINT('Ctrl Pts',(-10.0468807891092,18.1638733921006,79.257078036649));
#45271=CARTESIAN_POINT('Ctrl Pts',(-10.1339057616696,18.0287684620774,79.1549908365387));
#45272=CARTESIAN_POINT('Ctrl Pts',(-10.3514335308102,17.7609964409145,78.8743354225477));
#45273=CARTESIAN_POINT('Ctrl Pts',(-10.4832005944038,17.650192730897,78.6864655686667));
#45274=CARTESIAN_POINT('Ctrl Pts',(-10.6338951387459,17.5385627946702,78.3634796463819));
#45275=CARTESIAN_POINT('Ctrl Pts',(-10.6729371667049,17.5140590169286,78.2399649670483));
#45276=CARTESIAN_POINT('Ctrl Pts',(-10.692640786038,17.5014920111156,78.0771284470038));
#45277=CARTESIAN_POINT('Ctrl Pts',(-10.6950125628934,17.5,78.0386867639672));
#45278=CARTESIAN_POINT('Ctrl Pts',(-10.6950125628934,17.5,78.));
#45279=CARTESIAN_POINT('',(-0.69250628144669,17.5,95.3248490824925));
#45280=CARTESIAN_POINT('Ctrl Pts',(-0.692506281446693,17.5,95.3248490824925));
#45281=CARTESIAN_POINT('Ctrl Pts',(-0.739651283187984,17.5,95.2976299030462));
#45282=CARTESIAN_POINT('Ctrl Pts',(-0.783921069024338,17.502946735144,95.2666399401801));
#45283=CARTESIAN_POINT('Ctrl Pts',(-0.893496164763615,17.5181479027027,
95.1760997427212));
#45284=CARTESIAN_POINT('Ctrl Pts',(-0.952868520844795,17.5348232538744,
95.1123110174761));
#45285=CARTESIAN_POINT('Ctrl Pts',(-1.0757881096407,17.5875127881648,94.9553936265909));
#45286=CARTESIAN_POINT('Ctrl Pts',(-1.1350738927336,17.6285240662611,94.858714438747));
#45287=CARTESIAN_POINT('Ctrl Pts',(-1.27449989198037,17.7623087481876,94.6004969583169));
#45288=CARTESIAN_POINT('Ctrl Pts',(-1.34772601572953,17.879686489264,94.4253234714407));
#45289=CARTESIAN_POINT('Ctrl Pts',(-1.45881833757545,18.166627289437,94.1330107665224));
#45290=CARTESIAN_POINT('Ctrl Pts',(-1.49869633517117,18.3256026756651,94.0144578388582));
#45291=CARTESIAN_POINT('Ctrl Pts',(-1.54565821971146,18.6468724886464,93.8716044496407));
#45292=CARTESIAN_POINT('Ctrl Pts',(-1.55739293701455,18.797169501223,93.8341411336913));
#45293=CARTESIAN_POINT('Ctrl Pts',(-1.55959597242036,18.9686255097769,93.8271836955436));
#45294=CARTESIAN_POINT('Ctrl Pts',(-1.55969639024622,18.984327656238,93.8268664107545));
#45295=CARTESIAN_POINT('Ctrl Pts',(-1.55969639024622,19.,93.8268664107545));
#45296=CARTESIAN_POINT('Ctrl Pts',(1.0383798211071,19.,95.3268664107545));
#45297=CARTESIAN_POINT('Ctrl Pts',(1.0383798211071,18.9648000704089,95.3268664107545));
#45298=CARTESIAN_POINT('Ctrl Pts',(1.03674060554243,18.9294832054732,95.327228284536));
#45299=CARTESIAN_POINT('Ctrl Pts',(1.01957967822326,18.7461724891624,95.3310039597947));
#45300=CARTESIAN_POINT('Ctrl Pts',(0.977180926756438,18.604082341791,95.3404093141259));
#45301=CARTESIAN_POINT('Ctrl Pts',(0.831990480065218,18.3102983306063,95.3704789896338));
#45302=CARTESIAN_POINT('Ctrl Pts',(0.720572662835746,18.1669858887455,95.3926645032412));
#45303=CARTESIAN_POINT('Ctrl Pts',(0.39768224056495,17.8610717494634,95.4455561631698));
#45304=CARTESIAN_POINT('Ctrl Pts',(0.169339084394697,17.7272792212462,95.4746565277455));
#45305=CARTESIAN_POINT('Ctrl Pts',(-0.178116496062518,17.5873420162312,
95.4719940269684));
#45306=CARTESIAN_POINT('Ctrl Pts',(-0.313632679545349,17.5470806517564,
95.4606117044499));
#45307=CARTESIAN_POINT('Ctrl Pts',(-0.506413617508378,17.5125581835725,
95.4094260880585));
#45308=CARTESIAN_POINT('Ctrl Pts',(-0.566499372114017,17.5052303115316,
95.388073307207));
#45309=CARTESIAN_POINT('Ctrl Pts',(-0.647804466045143,17.5006516995771,
95.3494644005024));
#45310=CARTESIAN_POINT('Ctrl Pts',(-0.670382323171821,17.5,95.3376223557581));
#45311=CARTESIAN_POINT('Ctrl Pts',(-0.692506281446687,17.5,95.3248490824925));
#45312=CARTESIAN_POINT('Origin',(16.36,19.,65.7890418066394));
#45313=CARTESIAN_POINT('',(15.0609618943234,19.,65.0390418066394));
#45314=CARTESIAN_POINT('Origin',(2.25999999999999,19.,65.7890418066394));
#45315=CARTESIAN_POINT('',(0.960961894323336,19.,66.5390418066394));
#45316=CARTESIAN_POINT('Origin',(-4.79,19.,78.));
#45317=CARTESIAN_POINT('',(-4.79,19.,79.5));
#45318=CARTESIAN_POINT('Origin',(2.26,19.,90.2109581933606));
#45319=CARTESIAN_POINT('',(3.55903810567666,19.,90.9609581933606));
#45320=CARTESIAN_POINT('Origin',(16.36,19.,90.2109581933606));
#45321=CARTESIAN_POINT('',(17.6590381056767,19.,89.4609581933606));
#45322=CARTESIAN_POINT('Origin',(23.41,19.,78.));
#45323=CARTESIAN_POINT('',(23.41,19.,76.5));
#45324=CARTESIAN_POINT('Origin',(9.31,23.45,78.));
#45325=CARTESIAN_POINT('',(6.2075,23.5,78.));
#45326=CARTESIAN_POINT('',(6.2575,23.45,78.));
#45327=CARTESIAN_POINT('Origin',(9.31,23.5,78.));
#45328=CARTESIAN_POINT('Origin',(16.61,23.5,78.));
#45329=CARTESIAN_POINT('',(2.01,23.5,78.));
#45330=CARTESIAN_POINT('Origin',(9.31,23.5,78.));
#45331=CARTESIAN_POINT('Origin',(9.31,23.4,78.));
#45332=CARTESIAN_POINT('',(1.91,23.4,78.));
#45333=CARTESIAN_POINT('Origin',(9.31,14.15,78.));
#45334=CARTESIAN_POINT('',(2.01,14.05,78.));
#45335=CARTESIAN_POINT('Origin',(9.31,14.05,78.));
#45336=CARTESIAN_POINT('',(1.91,14.15,78.));
#45337=CARTESIAN_POINT('Origin',(12.4125,14.05,78.));
#45338=CARTESIAN_POINT('',(6.2075,14.05,78.));
#45339=CARTESIAN_POINT('Origin',(9.31,14.05,78.));
#45340=CARTESIAN_POINT('Origin',(9.31,14.1,78.));
#45341=CARTESIAN_POINT('',(6.2575,14.1,78.));
#70729=UNCERTAINTY_MEASURE_WITH_UNIT(LENGTH_MEASURE(0.001),#70758,
'DISTANCE_ACCURACY_VALUE',
'Maximum model space distance between geometric entities at asserted c
onnectivities');
#70740=UNCERTAINTY_MEASURE_WITH_UNIT(LENGTH_MEASURE(0.001),#70758,
'DISTANCE_ACCURACY_VALUE',
'Maximum model space distance between geometric entities at asserted c
onnectivities');
#70746=(
GEOMETRIC_REPRESENTATION_CONTEXT(3)
GLOBAL_UNCERTAINTY_ASSIGNED_CONTEXT((#70729))
GLOBAL_UNIT_ASSIGNED_CONTEXT((#70758,#70760,#70761))
REPRESENTATION_CONTEXT('','3D')
);
#70757=(
GEOMETRIC_REPRESENTATION_CONTEXT(3)
GLOBAL_UNCERTAINTY_ASSIGNED_CONTEXT((#70740))
GLOBAL_UNIT_ASSIGNED_CONTEXT((#70758,#70760,#70761))
REPRESENTATION_CONTEXT('','3D')
);
#70758=(
LENGTH_UNIT()
NAMED_UNIT(*)
SI_UNIT(.CENTI.,.METRE.)
);
#70760=(
NAMED_UNIT(*)
PLANE_ANGLE_UNIT()
SI_UNIT($,.RADIAN.)
);
#70761=(
NAMED_UNIT(*)
SI_UNIT($,.STERADIAN.)
SOLID_ANGLE_UNIT()
);
#70767=SHAPE_DEFINITION_REPRESENTATION(#70783,#70822);
#70783=PRODUCT_DEFINITION_SHAPE('',$,#70839);
#70822=SHAPE_REPRESENTATION('',(#27399),#70746);
#70833=PRODUCT_DEFINITION_CONTEXT('part definition',#70883,'design');
#70839=PRODUCT_DEFINITION('2026-10-19-02-55-51-279',
'07_Quick-Return_Handwheel_D456_6-Spoke',#70855,#70833);
#70855=PRODUCT_DEFINITION_FORMATION('',$,#70890);
#70883=APPLICATION_CONTEXT(
'Core Data for Automotive Mechanical Design Process');
#70884=PRODUCT_CONTEXT('part definition',#70883,'mechanical');
#70890=PRODUCT('2026-10-19-02-55-51-279',
'07_Quick-Return_Handwheel_D456_6-Spoke',$,(#70884));
#71027=COLOUR_RGB('Light Blue',0.38,0.62,0.78);
#71028=FILL_AREA_STYLE_COLOUR('',#71027);
#71029=FILL_AREA_STYLE('',(#71028));
#71030=SURFACE_STYLE_FILL_AREA(#71029);
#71031=SURFACE_SIDE_STYLE('',(#71030));
#71032=SURFACE_STYLE_USAGE(.BOTH.,#71031);
#71033=PRESENTATION_STYLE_ASSIGNMENT((#71032));
ENDSEC;
END-ISO-10303-21;
